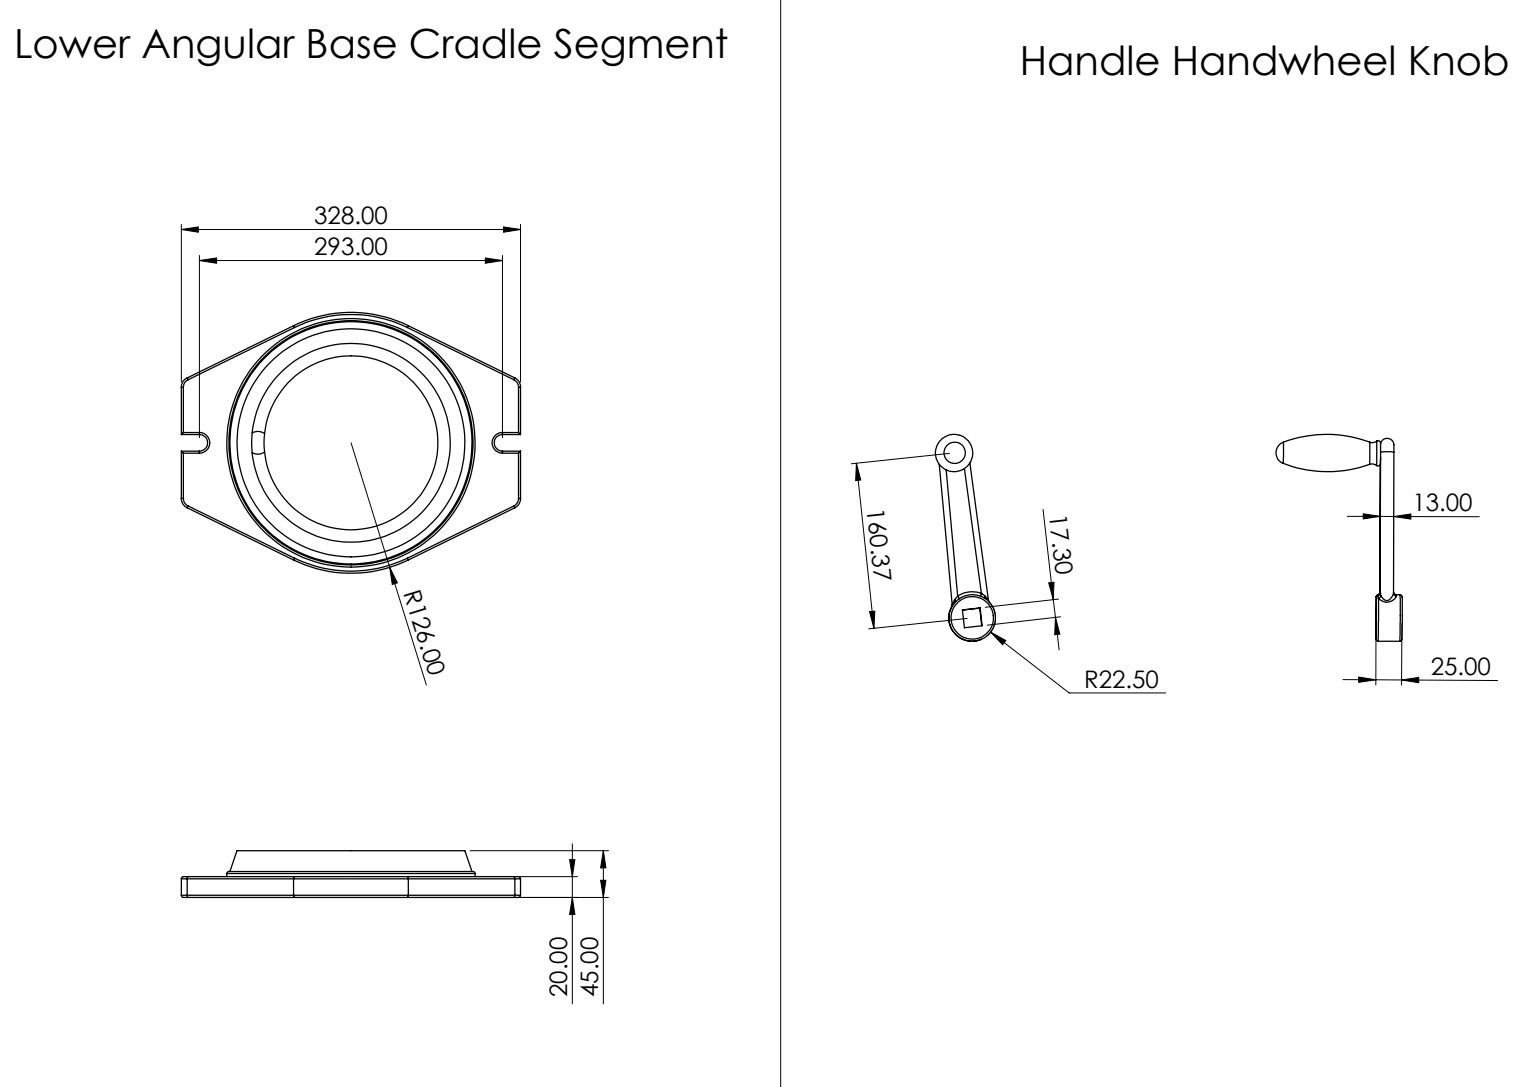
ISO-10303-21;
HEADER;
FILE_DESCRIPTION (('STEP AP214'),
    '1' );
FILE_NAME ('Lower Angular Base Cradle Segment.step',
    '2026-10-09T10:51:02',
    ( '' ),
    ( '' ),
    'SwSTEP 2.0',
    'SolidWorks 2026',
    '' );
FILE_SCHEMA (( 'AUTOMOTIVE_DESIGN' ));
ENDSEC;

DATA;
#11=AXIS2_PLACEMENT_3D ( 'NONE', #11203, #9587, #5900 ) ;
#14=ORIENTED_EDGE ( 'NONE', *, *, #14466, .T. ) ;
#36=VECTOR ( 'NONE', #11049, 1000.000000000000000 ) ;
#39=ORIENTED_EDGE ( 'NONE', *, *, #19350, .F. ) ;
#77=DIRECTION ( 'NONE',  ( 0.000000000000000000, 0.000000000000000000, -1.000000000000000000 ) ) ;
#83=DIRECTION ( 'NONE',  ( 0.000000000000000000, -1.000000000000000000, 0.000000000000000000 ) ) ;
#99=VERTEX_POINT ( 'NONE', #7105 ) ;
#118=EDGE_LOOP ( 'NONE', ( #17233, #4566 ) ) ;
#127=FACE_BOUND ( 'NONE', #21151, .T. ) ;
#139=ORIENTED_EDGE ( 'NONE', *, *, #21705, .T. ) ;
#155=EDGE_CURVE ( 'NONE', #11795, #1627, #509, .T. ) ;
#161=AXIS2_PLACEMENT_3D ( 'NONE', #9912, #15227, #6474 ) ;
#168=VERTEX_POINT ( 'NONE', #19161 ) ;
#170=EDGE_CURVE ( 'NONE', #168, #18579, #18934, .T. ) ;
#172=EDGE_CURVE ( 'NONE', #2811, #3408, #19534, .T. ) ;
#184=ORIENTED_EDGE ( 'NONE', *, *, #10599, .F. ) ;
#190=CIRCLE ( 'NONE', #9344, 2.000000000000000000 ) ;
#216=DIRECTION ( 'NONE',  ( 0.000000000000000000, 1.000000000000000000, -0.000000000000000000 ) ) ;
#237=DIRECTION ( 'NONE',  ( 0.000000000000000000, 0.000000000000000000, 1.000000000000000000 ) ) ;
#246=ORIENTED_EDGE ( 'NONE', *, *, #15979, .F. ) ;
#254=LINE ( 'NONE', #14055, #10043 ) ;
#259=DIRECTION ( 'NONE',  ( -0.000000000000000000, -1.000000000000000000, -0.000000000000000000 ) ) ;
#272=UNCERTAINTY_MEASURE_WITH_UNIT (LENGTH_MEASURE( 1.000000000000000082E-05 ), #22042, 'distance_accuracy_value', 'NONE');
#327=ORIENTED_EDGE ( 'NONE', *, *, #6954, .T. ) ;
#359=ORIENTED_EDGE ( 'NONE', *, *, #12423, .F. ) ;
#364=DIRECTION ( 'NONE',  ( -0.000000000000000000, -1.000000000000000000, 0.000000000000000000 ) ) ;
#443=VECTOR ( 'NONE', #5806, 1000.000000000000114 ) ;
#460=DIRECTION ( 'NONE',  ( 0.000000000000000000, 0.000000000000000000, 1.000000000000000000 ) ) ;
#465=AXIS2_PLACEMENT_3D ( 'NONE', #19858, #19338, #7694 ) ;
#466=AXIS2_PLACEMENT_3D ( 'NONE', #6505, #18462, #13187 ) ;
#468=DIRECTION ( 'NONE',  ( -0.000000000000000000, -1.000000000000000000, -0.000000000000000000 ) ) ;
#475=EDGE_CURVE ( 'NONE', #8008, #17969, #6839, .T. ) ;
#479=CIRCLE ( 'NONE', #8172, 10.00000000000001599 ) ;
#486=CARTESIAN_POINT ( 'NONE',  ( -164.0000000000000284, 19.17157287525381193, 8.000000000000019540 ) ) ;
#509=CIRCLE ( 'NONE', #21394, 8.000000000000003553 ) ;
#515=ORIENTED_EDGE ( 'NONE', *, *, #10366, .F. ) ;
#516=LINE ( 'NONE', #744, #20526 ) ;
#525=CARTESIAN_POINT ( 'NONE',  ( 163.9999999999992610, 1.999999999999998224, 53.76161406891480965 ) ) ;
#536=FACE_OUTER_BOUND ( 'NONE', #6630, .T. ) ;
#540=CARTESIAN_POINT ( 'NONE',  ( 161.9999999999998579, 0.000000000000000000, 10.00000000000220091 ) ) ;
#545=AXIS2_PLACEMENT_3D ( 'NONE', #10646, #3288, #5118 ) ;
#561=EDGE_CURVE ( 'NONE', #10233, #9740, #11615, .T. ) ;
#573=DIRECTION ( 'NONE',  ( 0.000000000000000000, -1.000000000000000000, 0.000000000000000000 ) ) ;
#576=CARTESIAN_POINT ( 'NONE',  ( -83.99999999999998579, 37.00000000000000711, 0.000000000000000000 ) ) ;
#585=EDGE_CURVE ( 'NONE', #7846, #1225, #20772, .T. ) ;
#605=DIRECTION ( 'NONE',  ( 0.000000000000000000, 0.000000000000000000, 1.000000000000000000 ) ) ;
#607=DIRECTION ( 'NONE',  ( -0.000000000000000000, -1.000000000000000000, 0.000000000000000000 ) ) ;
#614=ORIENTED_EDGE ( 'NONE', *, *, #21304, .F. ) ;
#619=ORIENTED_EDGE ( 'NONE', *, *, #6261, .F. ) ;
#620=ORIENTED_EDGE ( 'NONE', *, *, #15150, .T. ) ;
#632=EDGE_CURVE ( 'NONE', #17288, #1407, #18939, .T. ) ;
#636=EDGE_LOOP ( 'NONE', ( #1094, #22364, #825, #9647 ) ) ;
#643=CARTESIAN_POINT ( 'NONE',  ( -54.52327687265813694, 18.00000000000000355, 111.3697098814011781 ) ) ;
#654=DIRECTION ( 'NONE',  ( 0.000000000000000000, 0.000000000000000000, 1.000000000000000000 ) ) ;
#655=VECTOR ( 'NONE', #16102, 1000.000000000000000 ) ;
#660=CARTESIAN_POINT ( 'NONE',  ( 0.000000000000000000, 18.00000000000000355, 0.000000000000000000 ) ) ;
#669=EDGE_CURVE ( 'NONE', #4632, #17288, #3816, .T. ) ;
#671=ORIENTED_EDGE ( 'NONE', *, *, #11332, .T. ) ;
#673=AXIS2_PLACEMENT_3D ( 'NONE', #17290, #6819, #13736 ) ;
#688=CARTESIAN_POINT ( 'NONE',  ( 157.5176307659770885, 18.00000000000000355, -60.94675664190839370 ) ) ;
#695=CIRCLE ( 'NONE', #20840, 2.000000000000001332 ) ;
#706=ORIENTED_EDGE ( 'NONE', *, *, #11055, .F. ) ;
#724=VERTEX_POINT ( 'NONE', #1722 ) ;
#728=ORIENTED_EDGE ( 'NONE', *, *, #13180, .F. ) ;
#744=CARTESIAN_POINT ( 'NONE',  ( -146.5000000000000000, 20.00000000000000000, -7.999999999999981348 ) ) ;
#754=DIRECTION ( 'NONE',  ( -0.000000000000000000, -1.000000000000000000, -0.000000000000000000 ) ) ;
#756=DIRECTION ( 'NONE',  ( 0.8981428216242065554, 0.000000000000000000, 0.4397038457472354223 ) ) ;
#775=DIRECTION ( 'NONE',  ( 0.000000000000000000, 0.000000000000000000, -1.000000000000000000 ) ) ;
#777=DIRECTION ( 'NONE',  ( -1.000000000000000000, 0.000000000000000000, 0.000000000000000000 ) ) ;
#803=CARTESIAN_POINT ( 'NONE',  ( -164.0000000000000000, 18.00000000000000355, -53.76161406891256433 ) ) ;
#818=EDGE_CURVE ( 'NONE', #9599, #7572, #1748, .T. ) ;
#820=AXIS2_PLACEMENT_3D ( 'NONE', #8269, #17121, #15302 ) ;
#822=VERTEX_POINT ( 'NONE', #9641 ) ;
#825=ORIENTED_EDGE ( 'NONE', *, *, #1784, .F. ) ;
#827=AXIS2_PLACEMENT_3D ( 'NONE', #21475, #11159, #4013 ) ;
#867=DIRECTION ( 'NONE',  ( -0.8981428216242088869, 0.000000000000000000, 0.4397038457472309814 ) ) ;
#874=DIRECTION ( 'NONE',  ( 0.000000000000000000, 0.000000000000000000, -1.000000000000000000 ) ) ;
#893=DIRECTION ( 'NONE',  ( -0.000000000000000000, -1.000000000000000000, -0.000000000000000000 ) ) ;
#912=VECTOR ( 'NONE', #893, 1000.000000000000000 ) ;
#918=DIRECTION ( 'NONE',  ( 0.000000000000000000, -0.000000000000000000, 1.000000000000000000 ) ) ;
#924=LINE ( 'NONE', #16674, #12690 ) ;
#927=CARTESIAN_POINT ( 'NONE',  ( 1.236893267138826732E-14, 0.000000000000000000, 101.0000000000000000 ) ) ;
#955=DIRECTION ( 'NONE',  ( -0.000000000000000000, -1.000000000000000000, 0.000000000000000000 ) ) ;
#957=CARTESIAN_POINT ( 'NONE',  ( 162.0000000000000000, 1.999999999999998224, -2.262479907570350717E-12 ) ) ;
#966=CARTESIAN_POINT ( 'NONE',  ( -154.0000000000000000, 20.00000000000000000, -53.76161406891256433 ) ) ;
#972=CIRCLE ( 'NONE', #7187, 124.0000000000000000 ) ;
#977=DIRECTION ( 'NONE',  ( 0.4397038457472313144, 0.000000000000000000, -0.8981428216242086648 ) ) ;
#979=VERTEX_POINT ( 'NONE', #20950 ) ;
#982=ORIENTED_EDGE ( 'NONE', *, *, #22653, .T. ) ;
#1014=FACE_OUTER_BOUND ( 'NONE', #13248, .T. ) ;
#1018=VERTEX_POINT ( 'NONE', #4625 ) ;
#1025=DIRECTION ( 'NONE',  ( -1.000000000000000000, -0.000000000000000000, 9.912705577010318154E-17 ) ) ;
#1036=EDGE_LOOP ( 'NONE', ( #10873, #8707, #4402, #327 ) ) ;
#1044=DIRECTION ( 'NONE',  ( 0.000000000000000000, 1.000000000000000000, -0.000000000000000000 ) ) ;
#1047=DIRECTION ( 'NONE',  ( 0.000000000000000000, 0.000000000000000000, -1.000000000000000000 ) ) ;
#1050=DIRECTION ( 'NONE',  ( 0.8981428216242087759, -0.000000000000000000, -0.4397038457472309259 ) ) ;
#1052=DIRECTION ( 'NONE',  ( -0.000000000000000000, -1.000000000000000000, -0.000000000000000000 ) ) ;
#1055=DIRECTION ( 'NONE',  ( 1.458023040593674599E-16, 0.000000000000000000, 1.000000000000000000 ) ) ;
#1071=CYLINDRICAL_SURFACE ( 'NONE', #2276, 2.000000000000000000 ) ;
#1079=VECTOR ( 'NONE', #1276, 1000.000000000000000 ) ;
#1085=EDGE_CURVE ( 'NONE', #16346, #2665, #17059, .T. ) ;
#1090=CARTESIAN_POINT ( 'NONE',  ( 1.028703311283776507E-14, 45.00000000000000711, 83.99999999999998579 ) ) ;
#1094=ORIENTED_EDGE ( 'NONE', *, *, #6261, .T. ) ;
#1098=EDGE_CURVE ( 'NONE', #11124, #4632, #21172, .T. ) ;
#1102=ORIENTED_EDGE ( 'NONE', *, *, #1917, .T. ) ;
#1114=AXIS2_PLACEMENT_3D ( 'NONE', #8137, #15168, #22120 ) ;
#1154=CARTESIAN_POINT ( 'NONE',  ( -162.0000000000000000, 18.00000000000000355, -53.76161406891256433 ) ) ;
#1169=DIRECTION ( 'NONE',  ( -1.000000000000000000, 0.000000000000000000, 0.000000000000000000 ) ) ;
#1180=DIRECTION ( 'NONE',  ( -1.000000000000000000, 0.000000000000000000, 1.458023040593674599E-16 ) ) ;
#1181=CARTESIAN_POINT ( 'NONE',  ( 0.000000000000000000, 23.00000000000000000, 0.000000000000000000 ) ) ;
#1184=AXIS2_PLACEMENT_3D ( 'NONE', #9333, #5876, #12914 ) ;
#1185=DIRECTION ( 'NONE',  ( 0.000000000000000000, 0.000000000000000000, 1.000000000000000000 ) ) ;
#1192=CARTESIAN_POINT ( 'NONE',  ( 161.9999999999992610, 0.000000000000000000, 53.76161406891478123 ) ) ;
#1213=DIRECTION ( 'NONE',  ( -2.664535259100375697E-15, 0.000000000000000000, 1.000000000000000000 ) ) ;
#1214=CYLINDRICAL_SURFACE ( 'NONE', #18032, 2.000000000000001776 ) ;
#1225=VERTEX_POINT ( 'NONE', #3689 ) ;
#1241=EDGE_CURVE ( 'NONE', #1225, #14037, #18248, .T. ) ;
#1254=AXIS2_PLACEMENT_3D ( 'NONE', #3148, #17173, #10064 ) ;
#1269=DIRECTION ( 'NONE',  ( 2.449293598294706414E-16, 0.000000000000000000, 1.000000000000000000 ) ) ;
#1270=VECTOR ( 'NONE', #20131, 1000.000000000000000 ) ;
#1276=DIRECTION ( 'NONE',  ( -1.396592535537253658E-14, 0.000000000000000000, -1.000000000000000000 ) ) ;
#1282=ORIENTED_EDGE ( 'NONE', *, *, #11887, .F. ) ;
#1286=CARTESIAN_POINT ( 'NONE',  ( 54.52327687265659506, 20.00000000000000000, -111.3697098814019455 ) ) ;
#1288=VERTEX_POINT ( 'NONE', #2323 ) ;
#1296=CIRCLE ( 'NONE', #3486, 120.0000000000000000 ) ;
#1299=ADVANCED_FACE ( 'NONE', ( #19872 ), #18518, .F. ) ;
#1309=STYLED_ITEM ( 'NONE', ( #15085 ), #9845 ) ;
#1336=DIRECTION ( 'NONE',  ( 3.552713678800500929E-15, 0.000000000000000000, 1.000000000000000000 ) ) ;
#1339=DIRECTION ( 'NONE',  ( 1.000000000000000000, 0.000000000000000000, 1.372099599554301422E-14 ) ) ;
#1344=DIRECTION ( 'NONE',  ( -0.000000000000000000, -1.000000000000000000, -0.000000000000000000 ) ) ;
#1348=DIRECTION ( 'NONE',  ( 0.000000000000000000, 0.000000000000000000, -1.000000000000000000 ) ) ;
#1349=EDGE_CURVE ( 'NONE', #15641, #4119, #16444, .T. ) ;
#1350=ORIENTED_EDGE ( 'NONE', *, *, #13991, .F. ) ;
#1367=DIRECTION ( 'NONE',  ( 1.000000000000000000, -0.000000000000000000, -1.458023040593674599E-16 ) ) ;
#1375=DIRECTION ( 'NONE',  ( -0.000000000000000000, -1.000000000000000000, 0.000000000000000000 ) ) ;
#1380=CARTESIAN_POINT ( 'NONE',  ( 54.52327687265660927, 20.00000000000000000, 111.3697098814019029 ) ) ;
#1389=CARTESIAN_POINT ( 'NONE',  ( -164.0000000000000000, 18.00000000000000355, 0.000000000000000000 ) ) ;
#1392=ORIENTED_EDGE ( 'NONE', *, *, #10556, .F. ) ;
#1395=DIRECTION ( 'NONE',  ( 1.000000000000000000, 0.000000000000000000, 0.000000000000000000 ) ) ;
#1398=DIRECTION ( 'NONE',  ( 0.000000000000000000, 0.000000000000000000, -1.000000000000000000 ) ) ;
#1401=ORIENTED_EDGE ( 'NONE', *, *, #1478, .F. ) ;
#1407=VERTEX_POINT ( 'NONE', #22369 ) ;
#1431=EDGE_CURVE ( 'NONE', #1288, #17029, #10349, .T. ) ;
#1439=CIRCLE ( 'NONE', #6192, 78.99999999999998579 ) ;
#1440=ORIENTED_EDGE ( 'NONE', *, *, #17648, .T. ) ;
#1442=FACE_OUTER_BOUND ( 'NONE', #4234, .T. ) ;
#1443=DIRECTION ( 'NONE',  ( -0.000000000000000000, -1.000000000000000000, 0.000000000000000000 ) ) ;
#1478=EDGE_CURVE ( 'NONE', #9760, #979, #10929, .T. ) ;
#1501=EDGE_LOOP ( 'NONE', ( #17646, #17489, #7558, #20601, #8372, #14963, #15263, #20562, #9434, #13836, #9394, #3686, #8049, #16135, #18646, #21048, #4801, #16875, #2262, #19730, #15751 ) ) ;
#1519=AXIS2_PLACEMENT_3D ( 'NONE', #9593, #754, #11427 ) ;
#1522=EDGE_LOOP ( 'NONE', ( #6462, #16819, #9996, #12609 ) ) ;
#1523=EDGE_CURVE ( 'NONE', #9064, #5658, #4596, .T. ) ;
#1532=VERTEX_POINT ( 'NONE', #21232 ) ;
#1536=DIRECTION ( 'NONE',  ( 0.8981428216242028917, -0.000000000000000000, 0.4397038457472429718 ) ) ;
#1545=ORIENTED_EDGE ( 'NONE', *, *, #2061, .T. ) ;
#1550=VECTOR ( 'NONE', #4109, 1000.000000000000114 ) ;
#1551=EDGE_CURVE ( 'NONE', #9056, #6260, #1727, .T. ) ;
#1552=CARTESIAN_POINT ( 'NONE',  ( 0.000000000000000000, 25.00000000000000000, 0.000000000000000000 ) ) ;
#1554=PLANE ( 'NONE',  #3802 ) ;
#1558=CARTESIAN_POINT ( 'NONE',  ( 163.1715728752537018, 20.00000000000000355, -8.828427124748447596 ) ) ;
#1566=DIRECTION ( 'NONE',  ( 0.000000000000000000, 1.000000000000000000, 0.000000000000000000 ) ) ;
#1573=VECTOR ( 'NONE', #11501, 1000.000000000000000 ) ;
#1579=EDGE_LOOP ( 'NONE', ( #18293, #4104, #6095, #706 ) ) ;
#1580=CARTESIAN_POINT ( 'NONE',  ( 55.40268456415107323, 20.00000000000000000, -113.1659955246503557 ) ) ;
#1590=DIRECTION ( 'NONE',  ( 0.000000000000000000, 0.000000000000000000, 1.000000000000000000 ) ) ;
#1591=CARTESIAN_POINT ( 'NONE',  ( 157.5176307659770885, 20.00000000000000000, -60.94675664190840081 ) ) ;
#1604=ORIENTED_EDGE ( 'NONE', *, *, #10918, .T. ) ;
#1617=DIRECTION ( 'NONE',  ( 0.8981428216242088869, -0.000000000000000000, 0.4397038457472307593 ) ) ;
#1622=DIRECTION ( 'NONE',  ( 0.000000000000000000, -1.000000000000000000, 0.000000000000000000 ) ) ;
#1627=VERTEX_POINT ( 'NONE', #2968 ) ;
#1640=CARTESIAN_POINT ( 'NONE',  ( 0.000000000000000000, 45.00000000000000711, 0.000000000000000000 ) ) ;
#1660=CARTESIAN_POINT ( 'NONE',  ( -157.5176307659779411, 0.000000000000000000, 60.94675664190622655 ) ) ;
#1685=DIRECTION ( 'NONE',  ( -0.8981428216242028917, -0.000000000000000000, -0.4397038457472429718 ) ) ;
#1687=CARTESIAN_POINT ( 'NONE',  ( 0.000000000000000000, 20.00000000000000000, 0.000000000000000000 ) ) ;
#1693=CYLINDRICAL_SURFACE ( 'NONE', #7075, 8.000000000000003553 ) ;
#1714=DIRECTION ( 'NONE',  ( 0.000000000000000000, 0.000000000000000000, 1.000000000000000000 ) ) ;
#1721=DIRECTION ( 'NONE',  ( 0.000000000000000000, 0.000000000000000000, 1.000000000000000000 ) ) ;
#1722=CARTESIAN_POINT ( 'NONE',  ( 0.000000000000000000, 29.00000000000000711, -78.99999999999998579 ) ) ;
#1727=LINE ( 'NONE', #3893, #20440 ) ;
#1730=FACE_OUTER_BOUND ( 'NONE', #6402, .T. ) ;
#1742=EDGE_LOOP ( 'NONE', ( #11477, #2679, #19385, #12838 ) ) ;
#1748=CIRCLE ( 'NONE', #16801, 10.99999999999999289 ) ;
#1774=DIRECTION ( 'NONE',  ( -0.000000000000000000, -1.000000000000000000, -0.000000000000000000 ) ) ;
#1776=EDGE_CURVE ( 'NONE', #19048, #15773, #9846, .T. ) ;
#1782=AXIS2_PLACEMENT_3D ( 'NONE', #17932, #2168, #5721 ) ;
#1784=EDGE_CURVE ( 'NONE', #10110, #15773, #14258, .T. ) ;
#1786=DIRECTION ( 'NONE',  ( 1.000000000000000000, 0.000000000000000000, 0.000000000000000000 ) ) ;
#1794=ORIENTED_EDGE ( 'NONE', *, *, #18920, .F. ) ;
#1806=AXIS2_PLACEMENT_3D ( 'NONE', #5627, #7469, #5505 ) ;
#1808=DIRECTION ( 'NONE',  ( 0.000000000000000000, -1.000000000000000000, 0.000000000000000000 ) ) ;
#1809=DIRECTION ( 'NONE',  ( 0.000000000000000000, 0.000000000000000000, 1.000000000000000000 ) ) ;
#1829=EDGE_LOOP ( 'NONE', ( #4335, #17107, #8899, #14315, #21275, #17558, #10360, #7844, #3415, #6564 ) ) ;
#1831=ORIENTED_EDGE ( 'NONE', *, *, #20609, .T. ) ;
#1842=CIRCLE ( 'NONE', #13223, 101.0000000000000000 ) ;
#1852=CARTESIAN_POINT ( 'NONE',  ( 54.52327687265658085, 20.00000000000000000, -111.3697098814019171 ) ) ;
#1873=ORIENTED_EDGE ( 'NONE', *, *, #12470, .F. ) ;
#1879=VERTEX_POINT ( 'NONE', #21086 ) ;
#1909=AXIS2_PLACEMENT_3D ( 'NONE', #9756, #18257, #14830 ) ;
#1917=EDGE_CURVE ( 'NONE', #5531, #19256, #2593, .T. ) ;
#1926=CARTESIAN_POINT ( 'NONE',  ( -157.5176307659779127, 20.00000000000000000, 60.94675664190624786 ) ) ;
#1936=ADVANCED_FACE ( 'NONE', ( #536 ), #9602, .T. ) ;
#1971=CIRCLE ( 'NONE', #19570, 10.00000000000001599 ) ;
#1972=ORIENTED_EDGE ( 'NONE', *, *, #18630, .F. ) ;
#1975=FACE_OUTER_BOUND ( 'NONE', #9307, .T. ) ;
#1978=DIRECTION ( 'NONE',  ( -0.000000000000000000, -0.000000000000000000, 1.000000000000000000 ) ) ;
#1980=ADVANCED_FACE ( 'NONE', ( #20604 ), #15249, .T. ) ;
#1982=ORIENTED_EDGE ( 'NONE', *, *, #1431, .F. ) ;
#1991=VERTEX_POINT ( 'NONE', #18883 ) ;
#2000=EDGE_LOOP ( 'NONE', ( #18719, #17410, #7375, #11157 ) ) ;
#2003=AXIS2_PLACEMENT_3D ( 'NONE', #9292, #4227, #460 ) ;
#2011=ADVANCED_FACE ( 'NONE', ( #1442 ), #8422, .T. ) ;
#2028=DIRECTION ( 'NONE',  ( 0.000000000000000000, 0.000000000000000000, -1.000000000000000000 ) ) ;
#2030=ORIENTED_EDGE ( 'NONE', *, *, #6944, .T. ) ;
#2034=ADVANCED_FACE ( 'NONE', ( #4971 ), #12001, .T. ) ;
#2061=EDGE_CURVE ( 'NONE', #10705, #9211, #22294, .T. ) ;
#2069=EDGE_CURVE ( 'NONE', #21740, #9403, #15804, .T. ) ;
#2089=ADVANCED_FACE ( 'NONE', ( #12577 ), #8646, .F. ) ;
#2096=DIRECTION ( 'NONE',  ( 0.000000000000000000, 0.000000000000000000, 1.000000000000000000 ) ) ;
#2101=LINE ( 'NONE', #1660, #12535 ) ;
#2103=ORIENTED_EDGE ( 'NONE', *, *, #18624, .T. ) ;
#2106=ORIENTED_EDGE ( 'NONE', *, *, #19715, .T. ) ;
#2130=CARTESIAN_POINT ( 'NONE',  ( 146.5000000000000000, 20.00000000000000000, -2.025191382850354537E-12 ) ) ;
#2134=VERTEX_POINT ( 'NONE', #8879 ) ;
#2137=PRODUCT_DEFINITION ( 'UNKNOWN', '', #8434, #18911 ) ;
#2153=ORIENTED_EDGE ( 'NONE', *, *, #21573, .T. ) ;
#2156=AXIS2_PLACEMENT_3D ( 'NONE', #8737, #13938, #14184 ) ;
#2168=DIRECTION ( 'NONE',  ( 0.000000000000000000, 1.000000000000000000, -0.000000000000000000 ) ) ;
#2184=LINE ( 'NONE', #21035, #3366 ) ;
#2207=AXIS2_PLACEMENT_3D ( 'NONE', #18108, #11544, #7746 ) ;
#2218=AXIS2_PLACEMENT_3D ( 'NONE', #6057, #13192, #15152 ) ;
#2223=DIRECTION ( 'NONE',  ( 0.000000000000000000, 0.000000000000000000, 1.000000000000000000 ) ) ;
#2224=CYLINDRICAL_SURFACE ( 'NONE', #10412, 2.000000000000004441 ) ;
#2239=EDGE_CURVE ( 'NONE', #3243, #7424, #19014, .T. ) ;
#2247=CIRCLE ( 'NONE', #11065, 2.000000000000000000 ) ;
#2261=DIRECTION ( 'NONE',  ( 0.000000000000000000, 1.000000000000000000, -0.000000000000000000 ) ) ;
#2262=ORIENTED_EDGE ( 'NONE', *, *, #10736, .T. ) ;
#2272=ORIENTED_EDGE ( 'NONE', *, *, #5577, .T. ) ;
#2276=AXIS2_PLACEMENT_3D ( 'NONE', #15101, #6359, #20355 ) ;
#2282=CARTESIAN_POINT ( 'NONE',  ( -158.3970384574724051, 18.00000000000000355, 62.74304228515463677 ) ) ;
#2293=DIRECTION ( 'NONE',  ( 0.4397038457472340900, 0.000000000000000000, -0.8981428216242072216 ) ) ;
#2297=CARTESIAN_POINT ( 'NONE',  ( -101.0000000000000000, 29.00000000000000355, 9.420035382405126825E-16 ) ) ;
#2307=CARTESIAN_POINT ( 'NONE',  ( -162.0000000000000000, 18.00000000000000355, 3.967855629237424480E-14 ) ) ;
#2316=AXIS2_PLACEMENT_3D ( 'NONE', #8607, #13906, #237 ) ;
#2323=CARTESIAN_POINT ( 'NONE',  ( 157.5176307659771169, 0.000000000000000000, 60.94675664190834397 ) ) ;
#2327=DIRECTION ( 'NONE',  ( 0.000000000000000000, 0.000000000000000000, -1.000000000000000000 ) ) ;
#2334=ORIENTED_EDGE ( 'NONE', *, *, #172, .F. ) ;
#2360=ORIENTED_EDGE ( 'NONE', *, *, #21029, .F. ) ;
#2382=AXIS2_PLACEMENT_3D ( 'NONE', #19722, #16437, #3785 ) ;
#2389=ORIENTED_EDGE ( 'NONE', *, *, #15150, .F. ) ;
#2412=VECTOR ( 'NONE', #10464, 1000.000000000000000 ) ;
#2426=ORIENTED_EDGE ( 'NONE', *, *, #4092, .T. ) ;
#2428=ORIENTED_EDGE ( 'NONE', *, *, #22655, .T. ) ;
#2456=DIRECTION ( 'NONE',  ( 0.000000000000000000, 0.000000000000000000, 1.000000000000000000 ) ) ;
#2461=CARTESIAN_POINT ( 'NONE',  ( 55.40268456415105902, 1.999999999999998224, -113.1659955246503699 ) ) ;
#2469=VERTEX_POINT ( 'NONE', #15654 ) ;
#2506=DIRECTION ( 'NONE',  ( -0.000000000000000000, -1.000000000000000000, 0.000000000000000000 ) ) ;
#2508=CIRCLE ( 'NONE', #7273, 83.99999999999998579 ) ;
#2514=DIRECTION ( 'NONE',  ( 0.000000000000000000, 1.000000000000000000, 0.000000000000000000 ) ) ;
#2528=ADVANCED_FACE ( 'NONE', ( #5844 ), #5968, .T. ) ;
#2532=ORIENTED_EDGE ( 'NONE', *, *, #12333, .F. ) ;
#2537=( BOUNDED_CURVE ( )  B_SPLINE_CURVE ( 3, ( #10708, #5746, #486, #3914 ),
 .UNSPECIFIED., .F., .T. ) 
 B_SPLINE_CURVE_WITH_KNOTS ( ( 4, 4 ),
 ( 1.570796326794896558, 3.141592653589793116 ),
 .UNSPECIFIED. ) 
 CURVE ( )  GEOMETRIC_REPRESENTATION_ITEM ( )  RATIONAL_B_SPLINE_CURVE ( ( 1.000000000000000000, 0.8047378541243649375, 0.8047378541243649375, 1.000000000000000000 ) ) 
 REPRESENTATION_ITEM ( '' )  );
#2544=ORIENTED_EDGE ( 'NONE', *, *, #19748, .T. ) ;
#2552=LINE ( 'NONE', #18082, #11928 ) ;
#2566=CIRCLE ( 'NONE', #4001, 96.00000000000000000 ) ;
#2573=FACE_OUTER_BOUND ( 'NONE', #1501, .T. ) ;
#2574=CARTESIAN_POINT ( 'NONE',  ( 146.4999999999998579, 0.000000000000000000, 10.00000000000199130 ) ) ;
#2581=AXIS2_PLACEMENT_3D ( 'NONE', #12804, #21729, #14437 ) ;
#2586=CARTESIAN_POINT ( 'NONE',  ( -55.40268456415264353, 1.999999999999998224, -113.1659955246495883 ) ) ;
#2593=LINE ( 'NONE', #7536, #20472 ) ;
#2595=VECTOR ( 'NONE', #19673, 1000.000000000000000 ) ;
#2616=CIRCLE ( 'NONE', #9940, 2.000000000000001776 ) ;
#2618=AXIS2_PLACEMENT_3D ( 'NONE', #22365, #10006, #4809 ) ;
#2620=CARTESIAN_POINT ( 'NONE',  ( 0.000000000000000000, 0.000000000000000000, 0.000000000000000000 ) ) ;
#2621=ADVANCED_FACE ( 'NONE', ( #4120 ), #3899, .T. ) ;
#2624=CARTESIAN_POINT ( 'NONE',  ( 146.4999999999998579, 0.000000000000000000, -10.00000000000202860 ) ) ;
#2633=DIRECTION ( 'NONE',  ( 0.000000000000000000, 1.000000000000000000, -0.000000000000000000 ) ) ;
#2645=DIRECTION ( 'NONE',  ( -1.000000000000000000, 0.000000000000000000, 0.000000000000000000 ) ) ;
#2650=EDGE_CURVE ( 'NONE', #9740, #19048, #18597, .T. ) ;
#2652=CARTESIAN_POINT ( 'NONE',  ( 0.000000000000000000, 18.00000000000000355, 0.000000000000000000 ) ) ;
#2658=FACE_OUTER_BOUND ( 'NONE', #17459, .T. ) ;
#2665=VERTEX_POINT ( 'NONE', #7812 ) ;
#2670=AXIS2_PLACEMENT_3D ( 'NONE', #6925, #14618, #7050 ) ;
#2674=DIRECTION ( 'NONE',  ( -0.000000000000000000, -1.000000000000000000, -0.000000000000000000 ) ) ;
#2679=ORIENTED_EDGE ( 'NONE', *, *, #19298, .F. ) ;
#2683=( BOUNDED_CURVE ( )  B_SPLINE_CURVE ( 3, ( #12861, #7800, #5720, #16550 ),
 .UNSPECIFIED., .F., .T. ) 
 B_SPLINE_CURVE_WITH_KNOTS ( ( 4, 4 ),
 ( 4.712388980384689674, 6.283185307179586232 ),
 .UNSPECIFIED. ) 
 CURVE ( )  GEOMETRIC_REPRESENTATION_ITEM ( )  RATIONAL_B_SPLINE_CURVE ( ( 1.000000000000000000, 0.8047378541243649375, 0.8047378541243649375, 1.000000000000000000 ) ) 
 REPRESENTATION_ITEM ( '' )  );
#2689=EDGE_CURVE ( 'NONE', #8292, #21383, #21901, .T. ) ;
#2690=FACE_OUTER_BOUND ( 'NONE', #20598, .T. ) ;
#2694=ORIENTED_EDGE ( 'NONE', *, *, #11745, .F. ) ;
#2696=FACE_OUTER_BOUND ( 'NONE', #21989, .T. ) ;
#2699=CARTESIAN_POINT ( 'NONE',  ( 54.52327687265658085, 18.00000000000000355, -111.3697098814019171 ) ) ;
#2707=LINE ( 'NONE', #6142, #1270 ) ;
#2711=ORIENTED_EDGE ( 'NONE', *, *, #16561, .F. ) ;
#2726=VECTOR ( 'NONE', #1050, 1000.000000000000114 ) ;
#2736=CARTESIAN_POINT ( 'NONE',  ( -164.0000000000000000, 20.00000000000000000, 0.000000000000000000 ) ) ;
#2739=FACE_OUTER_BOUND ( 'NONE', #22266, .T. ) ;
#2751=EDGE_CURVE ( 'NONE', #11917, #7779, #4721, .T. ) ;
#2767=CARTESIAN_POINT ( 'NONE',  ( 146.4999999999998863, 20.00000000000000000, 8.000000000001989520 ) ) ;
#2781=ORIENTED_EDGE ( 'NONE', *, *, #2751, .F. ) ;
#2794=EDGE_CURVE ( 'NONE', #22165, #19122, #2972, .T. ) ;
#2798=FACE_OUTER_BOUND ( 'NONE', #20156, .T. ) ;
#2811=VERTEX_POINT ( 'NONE', #1380 ) ;
#2812=DIRECTION ( 'NONE',  ( 0.000000000000000000, 0.000000000000000000, -1.000000000000000000 ) ) ;
#2832=EDGE_CURVE ( 'NONE', #5236, #822, #17460, .T. ) ;
#2837=VERTEX_POINT ( 'NONE', #14005 ) ;
#2846=FACE_OUTER_BOUND ( 'NONE', #10676, .T. ) ;
#2856=CARTESIAN_POINT ( 'NONE',  ( 0.000000000000000000, 37.00000000000000711, 0.000000000000000000 ) ) ;
#2859=DIRECTION ( 'NONE',  ( -1.000000000000000000, -0.000000000000000000, -0.000000000000000000 ) ) ;
#2865=ORIENTED_EDGE ( 'NONE', *, *, #17744, .F. ) ;
#2873=LINE ( 'NONE', #11721, #21268 ) ;
#2874=ORIENTED_EDGE ( 'NONE', *, *, #6944, .F. ) ;
#2892=EDGE_CURVE ( 'NONE', #12157, #8554, #13779, .T. ) ;
#2916=VERTEX_POINT ( 'NONE', #10442 ) ;
#2917=AXIS2_PLACEMENT_3D ( 'NONE', #1580, #20400, #13867 ) ;
#2919=CARTESIAN_POINT ( 'NONE',  ( -55.40268456415262932, 20.00000000000000000, 113.1659955246495883 ) ) ;
#2925=CARTESIAN_POINT ( 'NONE',  ( 0.000000000000000000, 0.000000000000000000, -78.99999999999998579 ) ) ;
#2928=FACE_OUTER_BOUND ( 'NONE', #1579, .T. ) ;
#2933=DIRECTION ( 'NONE',  ( -0.000000000000000000, -1.000000000000000000, -0.000000000000000000 ) ) ;
#2951=EDGE_CURVE ( 'NONE', #12157, #19445, #4786, .T. ) ;
#2955=VERTEX_POINT ( 'NONE', #5013 ) ;
#2961=CARTESIAN_POINT ( 'NONE',  ( 163.9999999999998863, 18.00000000000000355, 8.000000000002229328 ) ) ;
#2965=CARTESIAN_POINT ( 'NONE',  ( -164.0000000000000000, 20.00000000000000000, 53.76161406891260697 ) ) ;
#2968=CARTESIAN_POINT ( 'NONE',  ( -146.5000000000000000, 1.999999999999998224, 8.000000000000017764 ) ) ;
#2972=LINE ( 'NONE', #9987, #6926 ) ;
#2992=SURFACE_STYLE_USAGE ( .BOTH. , #9679 ) ;
#2995=AXIS2_PLACEMENT_3D ( 'NONE', #14715, #2633, #12992 ) ;
#3011=EDGE_CURVE ( 'NONE', #14045, #1288, #12477, .T. ) ;
#3013=AXIS2_PLACEMENT_3D ( 'NONE', #8562, #5101, #10300 ) ;
#3023=ORIENTED_EDGE ( 'NONE', *, *, #19180, .F. ) ;
#3030=VECTOR ( 'NONE', #19503, 1000.000000000000000 ) ;
#3032=ORIENTED_EDGE ( 'NONE', *, *, #13991, .T. ) ;
#3042=FACE_OUTER_BOUND ( 'NONE', #12897, .T. ) ;
#3048=AXIS2_PLACEMENT_3D ( 'NONE', #15582, #22532, #4864 ) ;
#3075=FACE_OUTER_BOUND ( 'NONE', #4265, .T. ) ;
#3085=CARTESIAN_POINT ( 'NONE',  ( 0.000000000000000000, 45.00000000000000711, -83.99999999999998579 ) ) ;
#3102=CARTESIAN_POINT ( 'NONE',  ( 0.000000000000000000, 0.000000000000000000, 0.000000000000000000 ) ) ;
#3128=ORIENTED_EDGE ( 'NONE', *, *, #1349, .F. ) ;
#3129=ORIENTED_EDGE ( 'NONE', *, *, #22301, .F. ) ;
#3135=( NAMED_UNIT ( * ) SI_UNIT ( $, .STERADIAN. ) SOLID_ANGLE_UNIT ( ) );
#3141=EDGE_CURVE ( 'NONE', #18838, #9416, #12211, .T. ) ;
#3148=CARTESIAN_POINT ( 'NONE',  ( -146.5000000000000000, 18.00000000000000355, 2.081668171172168513E-14 ) ) ;
#3149=EDGE_CURVE ( 'NONE', #10602, #22152, #21465, .T. ) ;
#3152=CARTESIAN_POINT ( 'NONE',  ( 1.445083222993876641E-14, 23.00000000000000000, -118.0000000000000000 ) ) ;
#3153=CARTESIAN_POINT ( 'NONE',  ( -90.00000000000000000, 45.00100000000000477, 10.99999999999999289 ) ) ;
#3178=DIRECTION ( 'NONE',  ( 0.000000000000000000, 0.000000000000000000, -1.000000000000000000 ) ) ;
#3180=DIRECTION ( 'NONE',  ( -1.000000000000000000, 0.000000000000000000, -1.362186893977296347E-14 ) ) ;
#3181=ADVANCED_FACE ( 'NONE', ( #19629 ), #11024, .T. ) ;
#3191=CARTESIAN_POINT ( 'NONE',  ( -55.40268456415265774, 18.00000000000000355, -113.1659955246495741 ) ) ;
#3196=CARTESIAN_POINT ( 'NONE',  ( -1.386679829960242619E-13, 20.00000000000000000, -9.999999999999994671 ) ) ;
#3217=ORIENTED_EDGE ( 'NONE', *, *, #1523, .F. ) ;
#3224=CARTESIAN_POINT ( 'NONE',  ( 146.4999999999998579, 20.00000000000000000, -10.00000000000202682 ) ) ;
#3243=VERTEX_POINT ( 'NONE', #18490 ) ;
#3246=ORIENTED_EDGE ( 'NONE', *, *, #6278, .F. ) ;
#3252=EDGE_CURVE ( 'NONE', #15219, #6364, #20313, .T. ) ;
#3254=VERTEX_POINT ( 'NONE', #11599 ) ;
#3267=ORIENTED_EDGE ( 'NONE', *, *, #818, .T. ) ;
#3276=CARTESIAN_POINT ( 'NONE',  ( 0.000000000000000000, 25.00000000000000000, -120.0000000000000000 ) ) ;
#3283=EDGE_CURVE ( 'NONE', #1879, #2134, #2566, .T. ) ;
#3288=DIRECTION ( 'NONE',  ( 0.000000000000000000, 1.000000000000000000, -0.000000000000000000 ) ) ;
#3298=DIRECTION ( 'NONE',  ( 0.4397038457472313144, 0.000000000000000000, -0.8981428216242086648 ) ) ;
#3310=CARTESIAN_POINT ( 'NONE',  ( 54.52327687265660927, 18.00000000000000355, 111.3697098814019029 ) ) ;
#3312=DIRECTION ( 'NONE',  ( 0.000000000000000000, 0.000000000000000000, -1.000000000000000000 ) ) ;
#3320=EDGE_LOOP ( 'NONE', ( #19313, #16483, #19262, #6872 ) ) ;
#3325=AXIS2_PLACEMENT_3D ( 'NONE', #11563, #18784, #12008 ) ;
#3348=VERTEX_POINT ( 'NONE', #3085 ) ;
#3349=DIRECTION ( 'NONE',  ( -0.000000000000000000, -1.000000000000000000, -0.000000000000000000 ) ) ;
#3350=AXIS2_PLACEMENT_3D ( 'NONE', #10883, #17909, #7433 ) ;
#3361=DIRECTION ( 'NONE',  ( 1.000000000000000000, 0.000000000000000000, 1.387778780781445676E-14 ) ) ;
#3363=DIRECTION ( 'NONE',  ( 0.000000000000000000, 1.000000000000000000, -0.000000000000000000 ) ) ;
#3366=VECTOR ( 'NONE', #5287, 1000.000000000000000 ) ;
#3368=AXIS2_PLACEMENT_3D ( 'NONE', #5009, #8347, #22339 ) ;
#3378=VECTOR ( 'NONE', #6174, 1000.000000000000000 ) ;
#3408=VERTEX_POINT ( 'NONE', #13883 ) ;
#3411=ORIENTED_EDGE ( 'NONE', *, *, #13888, .T. ) ;
#3415=ORIENTED_EDGE ( 'NONE', *, *, #12655, .F. ) ;
#3423=AXIS2_PLACEMENT_3D ( 'NONE', #20142, #7977, #4414 ) ;
#3432=DIRECTION ( 'NONE',  ( 1.000000000000000000, 0.000000000000000000, -9.912705577010318154E-17 ) ) ;
#3439=DIRECTION ( 'NONE',  ( -3.987059982602682030E-17, -0.9455185755993167351, -0.3255681544571568109 ) ) ;
#3450=PLANE ( 'NONE',  #2316 ) ;
#3451=DIRECTION ( 'NONE',  ( -0.4397038457472424167, 0.000000000000000000, -0.8981428216242032248 ) ) ;
#3485=EDGE_LOOP ( 'NONE', ( #7503, #21513, #17440, #14077 ) ) ;
#3486=AXIS2_PLACEMENT_3D ( 'NONE', #1181, #16592, #20220 ) ;
#3492=ORIENTED_EDGE ( 'NONE', *, *, #10051, .F. ) ;
#3495=CARTESIAN_POINT ( 'NONE',  ( -154.0000000000000000, 0.000000000000000000, 53.76161406891259986 ) ) ;
#3496=CARTESIAN_POINT ( 'NONE',  ( 1.469576158976823671E-14, 23.00000000000000000, 120.0000000000000000 ) ) ;
#3529=VERTEX_POINT ( 'NONE', #21652 ) ;
#3546=CARTESIAN_POINT ( 'NONE',  ( 157.5176307659771169, 20.00000000000000000, 60.94675664190834397 ) ) ;
#3547=DIRECTION ( 'NONE',  ( 0.000000000000000000, 1.000000000000000000, -0.000000000000000000 ) ) ;
#3569=CARTESIAN_POINT ( 'NONE',  ( 161.9999999999998579, 0.000000000000000000, 10.00000000000220091 ) ) ;
#3596=EDGE_CURVE ( 'NONE', #7779, #21740, #21595, .T. ) ;
#3607=VECTOR ( 'NONE', #16039, 1000.000000000000000 ) ;
#3632=VECTOR ( 'NONE', #20078, 1000.000000000000000 ) ;
#3634=LINE ( 'NONE', #10647, #14284 ) ;
#3652=DIRECTION ( 'NONE',  ( 0.000000000000000000, 0.000000000000000000, 1.000000000000000000 ) ) ;
#3653=DIRECTION ( 'NONE',  ( 0.8981428216242027807, 0.000000000000000000, -0.4397038457472431938 ) ) ;
#3659=VERTEX_POINT ( 'NONE', #5756 ) ;
#3666=DIRECTION ( 'NONE',  ( 0.000000000000000000, 0.000000000000000000, 1.000000000000000000 ) ) ;
#3682=CARTESIAN_POINT ( 'NONE',  ( -1.386679829960242619E-13, 2.000000000000000000, -9.999999999999994671 ) ) ;
#3686=ORIENTED_EDGE ( 'NONE', *, *, #2069, .T. ) ;
#3689=CARTESIAN_POINT ( 'NONE',  ( 3.086109933851330151E-14, 1.999999999999998224, 126.0000000000000000 ) ) ;
#3734=EDGE_LOOP ( 'NONE', ( #9958, #4107 ) ) ;
#3738=ADVANCED_FACE ( 'NONE', ( #14876 ), #21817, .T. ) ;
#3743=EDGE_CURVE ( 'NONE', #11172, #2955, #20824, .T. ) ;
#3768=VECTOR ( 'NONE', #14937, 1000.000000000000114 ) ;
#3772=EDGE_LOOP ( 'NONE', ( #2103, #9863, #21778, #6767 ) ) ;
#3783=DIRECTION ( 'NONE',  ( 0.000000000000000000, 0.000000000000000000, -1.000000000000000000 ) ) ;
#3785=DIRECTION ( 'NONE',  ( 0.000000000000000000, 0.000000000000000000, 1.000000000000000000 ) ) ;
#3788=VECTOR ( 'NONE', #18661, 1000.000000000000000 ) ;
#3789=AXIS2_PLACEMENT_3D ( 'NONE', #15759, #10684, #5378 ) ;
#3798=ADVANCED_FACE ( 'NONE', ( #6671 ), #14248, .T. ) ;
#3802=AXIS2_PLACEMENT_3D ( 'NONE', #10510, #7274, #7170 ) ;
#3809=ORIENTED_EDGE ( 'NONE', *, *, #2794, .F. ) ;
#3816=CIRCLE ( 'NONE', #16679, 8.000000000000003553 ) ;
#3832=DIRECTION ( 'NONE',  ( 1.000000000000000000, 0.000000000000000000, -1.387778780781445833E-14 ) ) ;
#3835=ORIENTED_EDGE ( 'NONE', *, *, #3149, .T. ) ;
#3862=ORIENTED_EDGE ( 'NONE', *, *, #3596, .F. ) ;
#3880=ADVANCED_FACE ( 'NONE', ( #13526 ), #20839, .T. ) ;
#3893=CARTESIAN_POINT ( 'NONE',  ( 55.40268456415105902, 20.00000000000000000, -113.1659955246503699 ) ) ;
#3899=CYLINDRICAL_SURFACE ( 'NONE', #3982, 2.000000000000001332 ) ;
#3903=ORIENTED_EDGE ( 'NONE', *, *, #3283, .F. ) ;
#3906=LINE ( 'NONE', #14270, #21683 ) ;
#3908=CARTESIAN_POINT ( 'NONE',  ( 153.9999999999992610, 18.00000000000000355, -53.76161406891471017 ) ) ;
#3911=ORIENTED_EDGE ( 'NONE', *, *, #6131, .F. ) ;
#3914=CARTESIAN_POINT ( 'NONE',  ( -164.0000000000000000, 18.00000000000000355, 8.000000000000019540 ) ) ;
#3937=VERTEX_POINT ( 'NONE', #13857 ) ;
#3967=DIRECTION ( 'NONE',  ( 0.4397038457472424167, 0.000000000000000000, -0.8981428216242032248 ) ) ;
#3982=AXIS2_PLACEMENT_3D ( 'NONE', #9058, #11260, #18269 ) ;
#3989=FACE_OUTER_BOUND ( 'NONE', #10763, .T. ) ;
#3994=ORIENTED_EDGE ( 'NONE', *, *, #17938, .T. ) ;
#4001=AXIS2_PLACEMENT_3D ( 'NONE', #2856, #15179, #18821 ) ;
#4002=ORIENTED_EDGE ( 'NONE', *, *, #21675, .T. ) ;
#4010=EDGE_LOOP ( 'NONE', ( #2428, #19590, #9387, #16670 ) ) ;
#4013=DIRECTION ( 'NONE',  ( 0.000000000000000000, 0.000000000000000000, 1.000000000000000000 ) ) ;
#4024=DIRECTION ( 'NONE',  ( 0.000000000000000000, 1.000000000000000000, -0.000000000000000000 ) ) ;
#4042=CARTESIAN_POINT ( 'NONE',  ( -146.5000000000000000, 1.999999999999998224, -7.999999999999981348 ) ) ;
#4045=ADVANCED_FACE ( 'NONE', ( #6254 ), #17189, .T. ) ;
#4052=CARTESIAN_POINT ( 'NONE',  ( -162.0000000000000000, 0.000000000000000000, -53.76161406891256433 ) ) ;
#4064=ORIENTED_EDGE ( 'NONE', *, *, #13445, .F. ) ;
#4075=CARTESIAN_POINT ( 'NONE',  ( 163.9999999999998295, 0.8284271247461892917, -8.000000000002268408 ) ) ;
#4088=ORIENTED_EDGE ( 'NONE', *, *, #17676, .F. ) ;
#4092=EDGE_CURVE ( 'NONE', #822, #10707, #695, .T. ) ;
#4102=LINE ( 'NONE', #5479, #3030 ) ;
#4104=ORIENTED_EDGE ( 'NONE', *, *, #9891, .F. ) ;
#4107=ORIENTED_EDGE ( 'NONE', *, *, #4169, .F. ) ;
#4109=DIRECTION ( 'NONE',  ( 0.8981428216242087759, -0.000000000000000000, -0.4397038457472309259 ) ) ;
#4115=DIRECTION ( 'NONE',  ( 0.000000000000000000, 1.000000000000000000, -0.000000000000000000 ) ) ;
#4116=CIRCLE ( 'NONE', #8892, 2.000000000000001776 ) ;
#4119=VERTEX_POINT ( 'NONE', #2586 ) ;
#4120=FACE_OUTER_BOUND ( 'NONE', #13840, .T. ) ;
#4141=DIRECTION ( 'NONE',  ( 0.000000000000000000, 0.000000000000000000, -1.000000000000000000 ) ) ;
#4155=AXIS2_PLACEMENT_3D ( 'NONE', #3682, #15780, #14403 ) ;
#4158=AXIS2_PLACEMENT_3D ( 'NONE', #12119, #12464, #8882 ) ;
#4168=CARTESIAN_POINT ( 'NONE',  ( 0.000000000000000000, 29.00000000000000355, -101.0000000000000000 ) ) ;
#4169=EDGE_CURVE ( 'NONE', #9064, #3348, #2508, .T. ) ;
#4175=AXIS2_PLACEMENT_3D ( 'NONE', #10513, #3547, #10673 ) ;
#4198=CARTESIAN_POINT ( 'NONE',  ( 163.9999999999992610, 18.00000000000000355, 53.76161406891480965 ) ) ;
#4205=AXIS2_PLACEMENT_3D ( 'NONE', #14508, #5729, #11029 ) ;
#4227=DIRECTION ( 'NONE',  ( 0.000000000000000000, 1.000000000000000000, -0.000000000000000000 ) ) ;
#4231=ORIENTED_EDGE ( 'NONE', *, *, #13180, .T. ) ;
#4233=DIRECTION ( 'NONE',  ( 0.4397038457472424167, 0.000000000000000000, 0.8981428216242032248 ) ) ;
#4234=EDGE_LOOP ( 'NONE', ( #5445, #11256, #17197, #20029 ) ) ;
#4239=CIRCLE ( 'NONE', #21836, 10.99999999999999289 ) ;
#4242=EDGE_CURVE ( 'NONE', #14514, #9599, #6234, .T. ) ;
#4247=DIRECTION ( 'NONE',  ( 0.000000000000000000, 0.000000000000000000, 1.000000000000000000 ) ) ;
#4252=FACE_OUTER_BOUND ( 'NONE', #5112, .T. ) ;
#4257=DIRECTION ( 'NONE',  ( -1.000000000000000000, 0.000000000000000000, 2.449293598294706414E-16 ) ) ;
#4258=FACE_OUTER_BOUND ( 'NONE', #14598, .T. ) ;
#4265=EDGE_LOOP ( 'NONE', ( #6241, #9467, #18304, #5417 ) ) ;
#4268=( BOUNDED_CURVE ( )  B_SPLINE_CURVE ( 3, ( #21207, #9263, #9024, #14578 ),
 .UNSPECIFIED., .F., .T. ) 
 B_SPLINE_CURVE_WITH_KNOTS ( ( 4, 4 ),
 ( 3.141592653589793116, 4.712388980384689674 ),
 .UNSPECIFIED. ) 
 CURVE ( )  GEOMETRIC_REPRESENTATION_ITEM ( )  RATIONAL_B_SPLINE_CURVE ( ( 1.000000000000000000, 0.8047378541243649375, 0.8047378541243649375, 1.000000000000000000 ) ) 
 REPRESENTATION_ITEM ( '' )  );
#4290=AXIS2_PLACEMENT_3D ( 'NONE', #13494, #3361, #6802 ) ;
#4315=AXIS2_PLACEMENT_3D ( 'NONE', #10236, #22267, #1185 ) ;
#4327=ORIENTED_EDGE ( 'NONE', *, *, #17265, .F. ) ;
#4329=ORIENTED_EDGE ( 'NONE', *, *, #16427, .F. ) ;
#4335=ORIENTED_EDGE ( 'NONE', *, *, #9920, .F. ) ;
#4338=EDGE_CURVE ( 'NONE', #7424, #7803, #15375, .T. ) ;
#4342=DIRECTION ( 'NONE',  ( 0.000000000000000000, 0.000000000000000000, -1.000000000000000000 ) ) ;
#4351=FACE_OUTER_BOUND ( 'NONE', #6537, .T. ) ;
#4354=CARTESIAN_POINT ( 'NONE',  ( 0.000000000000000000, 29.00000000000000711, 0.000000000000000000 ) ) ;
#4356=ORIENTED_EDGE ( 'NONE', *, *, #18920, .T. ) ;
#4366=DIRECTION ( 'NONE',  ( 8.881784197001252323E-16, 0.000000000000000000, 1.000000000000000000 ) ) ;
#4370=DIRECTION ( 'NONE',  ( -0.000000000000000000, 0.000000000000000000, 1.000000000000000000 ) ) ;
#4371=ADVANCED_FACE ( 'NONE', ( #19985 ), #11274, .F. ) ;
#4378=ORIENTED_EDGE ( 'NONE', *, *, #6433, .F. ) ;
#4379=AXIS2_PLACEMENT_3D ( 'NONE', #9944, #4747, #10067 ) ;
#4402=ORIENTED_EDGE ( 'NONE', *, *, #13888, .F. ) ;
#4407=ORIENTED_EDGE ( 'NONE', *, *, #14925, .T. ) ;
#4413=EDGE_CURVE ( 'NONE', #9954, #10082, #19732, .T. ) ;
#4414=DIRECTION ( 'NONE',  ( -0.4397038457472493556, 0.000000000000000000, -0.8981428216241997831 ) ) ;
#4434=VECTOR ( 'NONE', #1685, 1000.000000000000114 ) ;
#4438=CARTESIAN_POINT ( 'NONE',  ( 161.9999999999998579, 20.00000000000000000, 10.00000000000220091 ) ) ;
#4448=AXIS2_PLACEMENT_3D ( 'NONE', #9926, #20713, #4963 ) ;
#4458=AXIS2_PLACEMENT_3D ( 'NONE', #13144, #13378, #16719 ) ;
#4464=AXIS2_PLACEMENT_3D ( 'NONE', #576, #12752, #3783 ) ;
#4471=CARTESIAN_POINT ( 'NONE',  ( 161.9999999999998863, 20.00000000000000000, 8.000000000002200906 ) ) ;
#4478=ORIENTED_EDGE ( 'NONE', *, *, #15979, .T. ) ;
#4482=DIRECTION ( 'NONE',  ( 0.000000000000000000, 1.000000000000000000, -0.000000000000000000 ) ) ;
#4484=AXIS2_PLACEMENT_3D ( 'NONE', #13520, #777, #16753 ) ;
#4492=DIRECTION ( 'NONE',  ( 0.000000000000000000, 0.000000000000000000, 1.000000000000000000 ) ) ;
#4499=CIRCLE ( 'NONE', #7443, 101.0000000000000000 ) ;
#4512=DIRECTION ( 'NONE',  ( -1.000000000000000000, 0.000000000000000000, -1.362186893977296347E-14 ) ) ;
#4524=ORIENTED_EDGE ( 'NONE', *, *, #15793, .F. ) ;
#4526=CIRCLE ( 'NONE', #21026, 126.0000000000000000 ) ;
#4533=DIRECTION ( 'NONE',  ( -0.000000000000000000, -1.000000000000000000, -0.000000000000000000 ) ) ;
#4553=AXIS2_PLACEMENT_3D ( 'NONE', #17931, #19623, #12753 ) ;
#4566=ORIENTED_EDGE ( 'NONE', *, *, #8797, .F. ) ;
#4568=DIRECTION ( 'NONE',  ( 1.372099599554306628E-14, -0.000000000000000000, -1.000000000000000000 ) ) ;
#4572=ADVANCED_FACE ( 'NONE', ( #21688 ), #19857, .T. ) ;
#4573=ORIENTED_EDGE ( 'NONE', *, *, #1098, .F. ) ;
#4578=ORIENTED_EDGE ( 'NONE', *, *, #12470, .T. ) ;
#4584=DIRECTION ( 'NONE',  ( 0.000000000000000000, -1.000000000000000000, 0.000000000000000000 ) ) ;
#4596=LINE ( 'NONE', #21014, #655 ) ;
#4597=CARTESIAN_POINT ( 'NONE',  ( -158.3970384574724335, 20.00000000000000000, -62.74304228515459414 ) ) ;
#4602=DIRECTION ( 'NONE',  ( -1.396592535537253658E-14, 0.000000000000000000, -1.000000000000000000 ) ) ;
#4615=ORIENTED_EDGE ( 'NONE', *, *, #1551, .T. ) ;
#4625=CARTESIAN_POINT ( 'NONE',  ( 0.000000000000000000, 37.00000000000000711, -78.99999999999998579 ) ) ;
#4628=ORIENTED_EDGE ( 'NONE', *, *, #1917, .F. ) ;
#4630=CARTESIAN_POINT ( 'NONE',  ( 158.3970384574715808, 18.00000000000000355, 62.74304228515676130 ) ) ;
#4632=VERTEX_POINT ( 'NONE', #12881 ) ;
#4635=ADVANCED_FACE ( 'NONE', ( #6086 ), #16354, .T. ) ;
#4636=EDGE_CURVE ( 'NONE', #7423, #9056, #6573, .T. ) ;
#4641=CARTESIAN_POINT ( 'NONE',  ( 163.9999999999998579, 0.000000000000000000, 10.00000000000222933 ) ) ;
#4646=CYLINDRICAL_SURFACE ( 'NONE', #16554, 10.99999999999999289 ) ;
#4663=CYLINDRICAL_SURFACE ( 'NONE', #13750, 96.00000000000000000 ) ;
#4665=ORIENTED_EDGE ( 'NONE', *, *, #14997, .F. ) ;
#4666=DIRECTION ( 'NONE',  ( 0.000000000000000000, -1.000000000000000000, 0.000000000000000000 ) ) ;
#4669=ADVANCED_FACE ( 'NONE', ( #8029 ), #21906, .T. ) ;
#4672=EDGE_CURVE ( 'NONE', #17969, #724, #1439, .T. ) ;
#4692=CARTESIAN_POINT ( 'NONE',  ( 0.000000000000000000, 37.00000000000000711, 0.000000000000000000 ) ) ;
#4700=DIRECTION ( 'NONE',  ( -1.000000000000000000, 0.000000000000000000, 1.396592535537260757E-14 ) ) ;
#4707=ADVANCED_FACE ( 'NONE', ( #2739 ), #6297, .T. ) ;
#4721=CIRCLE ( 'NONE', #12461, 2.000000000000001776 ) ;
#4731=( BOUNDED_CURVE ( )  B_SPLINE_CURVE ( 3, ( #20272, #20728, #1558, #18996 ),
 .UNSPECIFIED., .F., .T. ) 
 B_SPLINE_CURVE_WITH_KNOTS ( ( 4, 4 ),
 ( 0.000000000000000000, 1.570796326794896558 ),
 .UNSPECIFIED. ) 
 CURVE ( )  GEOMETRIC_REPRESENTATION_ITEM ( )  RATIONAL_B_SPLINE_CURVE ( ( 1.000000000000000000, 0.8047378541243649375, 0.8047378541243649375, 1.000000000000000000 ) ) 
 REPRESENTATION_ITEM ( '' )  );
#4738=VECTOR ( 'NONE', #13774, 1000.000000000000000 ) ;
#4747=DIRECTION ( 'NONE',  ( -1.000000000000000000, 0.000000000000000000, 1.458023040593674599E-16 ) ) ;
#4760=ORIENTED_EDGE ( 'NONE', *, *, #1478, .T. ) ;
#4765=DIRECTION ( 'NONE',  ( -1.000000000000000000, 0.000000000000000000, 0.000000000000000000 ) ) ;
#4774=EDGE_CURVE ( 'NONE', #5658, #15608, #15761, .T. ) ;
#4775=ORIENTED_EDGE ( 'NONE', *, *, #4774, .T. ) ;
#4779=DIRECTION ( 'NONE',  ( 0.000000000000000000, 0.000000000000000000, -1.000000000000000000 ) ) ;
#4786=LINE ( 'NONE', #2965, #4738 ) ;
#4790=ORIENTED_EDGE ( 'NONE', *, *, #7603, .T. ) ;
#4791=CARTESIAN_POINT ( 'NONE',  ( -1.362186893977295590E-13, 20.00000000000000000, 9.999999999999994671 ) ) ;
#4801=ORIENTED_EDGE ( 'NONE', *, *, #20623, .T. ) ;
#4805=ORIENTED_EDGE ( 'NONE', *, *, #585, .F. ) ;
#4809=DIRECTION ( 'NONE',  ( 1.000000000000000000, 0.000000000000000000, -1.387778780781444413E-14 ) ) ;
#4810=DIRECTION ( 'NONE',  ( 0.4397038457472354778, 0.000000000000000000, -0.8981428216242066664 ) ) ;
#4811=DIRECTION ( 'NONE',  ( 0.000000000000000000, 0.000000000000000000, 1.000000000000000000 ) ) ;
#4813=EDGE_CURVE ( 'NONE', #8554, #18838, #3634, .T. ) ;
#4818=ORIENTED_EDGE ( 'NONE', *, *, #18267, .F. ) ;
#4846=CARTESIAN_POINT ( 'NONE',  ( -146.5000000000000000, 0.000000000000000000, 2.081668171172168513E-14 ) ) ;
#4856=CIRCLE ( 'NONE', #466, 10.00000000000000355 ) ;
#4864=DIRECTION ( 'NONE',  ( 0.000000000000000000, 0.000000000000000000, 1.000000000000000000 ) ) ;
#4866=DIRECTION ( 'NONE',  ( 1.000000000000000000, -0.000000000000000000, 1.224646799147353207E-16 ) ) ;
#4879=CARTESIAN_POINT ( 'NONE',  ( 163.9999999999992610, 18.00000000000000355, -53.76161406891485228 ) ) ;
#4880=ORIENTED_EDGE ( 'NONE', *, *, #9948, .F. ) ;
#4890=CARTESIAN_POINT ( 'NONE',  ( 0.000000000000000000, 37.00000000000000711, 0.000000000000000000 ) ) ;
#4894=ORIENTED_EDGE ( 'NONE', *, *, #11683, .F. ) ;
#4898=ADVANCED_FACE ( 'NONE', ( #6416 ), #6846, .F. ) ;
#4919=CIRCLE ( 'NONE', #17806, 2.000000000000000000 ) ;
#4933=FACE_OUTER_BOUND ( 'NONE', #5937, .T. ) ;
#4934=CARTESIAN_POINT ( 'NONE',  ( 0.000000000000000000, 0.000000000000000000, -83.99999999999998579 ) ) ;
#4935=EDGE_LOOP ( 'NONE', ( #10831, #2532, #11587, #5031 ) ) ;
#4956=DIRECTION ( 'NONE',  ( -0.000000000000000000, -1.000000000000000000, -0.000000000000000000 ) ) ;
#4963=DIRECTION ( 'NONE',  ( 0.000000000000000000, 0.000000000000000000, 1.000000000000000000 ) ) ;
#4964=ORIENTED_EDGE ( 'NONE', *, *, #20279, .T. ) ;
#4971=FACE_OUTER_BOUND ( 'NONE', #19893, .T. ) ;
#4992=AXIS2_PLACEMENT_3D ( 'NONE', #4354, #18392, #19745 ) ;
#5000=CARTESIAN_POINT ( 'NONE',  ( -146.5000000000000000, 18.00000000000000355, 10.00000000000001599 ) ) ;
#5009=CARTESIAN_POINT ( 'NONE',  ( 161.9999999999992610, 2.000000000000000000, -53.76161406891482386 ) ) ;
#5011=ADVANCED_FACE ( 'NONE', ( #7298 ), #6957, .T. ) ;
#5013=CARTESIAN_POINT ( 'NONE',  ( -164.0000000000000000, 1.999999999999998224, -53.76161406891256433 ) ) ;
#5031=ORIENTED_EDGE ( 'NONE', *, *, #13304, .F. ) ;
#5057=DIRECTION ( 'NONE',  ( 0.000000000000000000, 0.000000000000000000, -1.000000000000000000 ) ) ;
#5066=AXIS2_PLACEMENT_3D ( 'NONE', #9910, #8510, #6571 ) ;
#5068=VERTEX_POINT ( 'NONE', #11328 ) ;
#5076=EDGE_LOOP ( 'NONE', ( #10172, #6110, #1794, #4329 ) ) ;
#5080=CARTESIAN_POINT ( 'NONE',  ( -90.00000000000000000, 29.00000000000000355, -10.99999999999999289 ) ) ;
#5085=DIRECTION ( 'NONE',  ( 0.000000000000000000, 0.000000000000000000, -1.000000000000000000 ) ) ;
#5093=AXIS2_PLACEMENT_3D ( 'NONE', #14340, #21311, #9372 ) ;
#5098=ORIENTED_EDGE ( 'NONE', *, *, #11887, .T. ) ;
#5101=DIRECTION ( 'NONE',  ( 0.000000000000000000, 1.000000000000000000, 0.000000000000000000 ) ) ;
#5112=EDGE_LOOP ( 'NONE', ( #5374, #7654, #17754, #8951 ) ) ;
#5118=DIRECTION ( 'NONE',  ( 0.000000000000000000, 0.000000000000000000, 1.000000000000000000 ) ) ;
#5139=EDGE_CURVE ( 'NONE', #7464, #9403, #18680, .T. ) ;
#5142=AXIS2_PLACEMENT_3D ( 'NONE', #10381, #7256, #2096 ) ;
#5150=TOROIDAL_SURFACE ( 'NONE', #3325, 8.000000000000014211, 2.000000000000000000 ) ;
#5183=CIRCLE ( 'NONE', #4448, 8.000000000000014211 ) ;
#5190=ORIENTED_EDGE ( 'NONE', *, *, #3011, .F. ) ;
#5191=CIRCLE ( 'NONE', #827, 2.000000000000001776 ) ;
#5193=ORIENTED_EDGE ( 'NONE', *, *, #5577, .F. ) ;
#5210=CARTESIAN_POINT ( 'NONE',  ( 0.000000000000000000, 1.999999999999998224, 0.000000000000000000 ) ) ;
#5218=EDGE_LOOP ( 'NONE', ( #13370, #671, #21765, #18069 ) ) ;
#5227=ORIENTED_EDGE ( 'NONE', *, *, #19350, .T. ) ;
#5236=VERTEX_POINT ( 'NONE', #22428 ) ;
#5240=DIRECTION ( 'NONE',  ( 0.000000000000000000, 0.000000000000000000, 1.000000000000000000 ) ) ;
#5242=CIRCLE ( 'NONE', #1254, 8.000000000000003553 ) ;
#5249=AXIS2_PLACEMENT_3D ( 'NONE', #18516, #15079, #20214 ) ;
#5259=DIRECTION ( 'NONE',  ( 0.000000000000000000, 0.000000000000000000, 1.000000000000000000 ) ) ;
#5266=CARTESIAN_POINT ( 'NONE',  ( 54.52327687265659506, 1.999999999999998224, 111.3697098814018744 ) ) ;
#5272=DIRECTION ( 'NONE',  ( 0.000000000000000000, 0.000000000000000000, -1.000000000000000000 ) ) ;
#5274=ORIENTED_EDGE ( 'NONE', *, *, #17991, .F. ) ;
#5287=DIRECTION ( 'NONE',  ( -0.000000000000000000, -1.000000000000000000, -0.000000000000000000 ) ) ;
#5291=ADVANCED_FACE ( 'NONE', ( #14278 ), #14684, .T. ) ;
#5293=DIRECTION ( 'NONE',  ( -0.000000000000000000, -1.000000000000000000, -0.000000000000000000 ) ) ;
#5308=LINE ( 'NONE', #12348, #7014 ) ;
#5368=VECTOR ( 'NONE', #8036, 1000.000000000000000 ) ;
#5370=DIRECTION ( 'NONE',  ( -0.000000000000000000, -1.000000000000000000, -0.000000000000000000 ) ) ;
#5374=ORIENTED_EDGE ( 'NONE', *, *, #2751, .T. ) ;
#5378=DIRECTION ( 'NONE',  ( 0.000000000000000000, 0.000000000000000000, 1.000000000000000000 ) ) ;
#5383=ORIENTED_EDGE ( 'NONE', *, *, #6810, .F. ) ;
#5387=EDGE_CURVE ( 'NONE', #8011, #7061, #2873, .T. ) ;
#5388=ORIENTED_EDGE ( 'NONE', *, *, #669, .T. ) ;
#5414=ADVANCED_FACE ( 'NONE', ( #4252 ), #8777, .T. ) ;
#5417=ORIENTED_EDGE ( 'NONE', *, *, #15568, .F. ) ;
#5421=APPLICATION_CONTEXT ( 'automotive_design' ) ;
#5436=AXIS2_PLACEMENT_3D ( 'NONE', #1552, #8538, #13841 ) ;
#5445=ORIENTED_EDGE ( 'NONE', *, *, #16605, .T. ) ;
#5455=ORIENTED_EDGE ( 'NONE', *, *, #16572, .T. ) ;
#5468=SHAPE_REPRESENTATION ( 'Lower Angular Base Cradle Segment', ( #6292 ), #7758 ) ;
#5471=ORIENTED_EDGE ( 'NONE', *, *, #20609, .F. ) ;
#5479=CARTESIAN_POINT ( 'NONE',  ( 1.175660927181459158E-14, 0.000000000000000000, 96.00000000000000000 ) ) ;
#5487=ORIENTED_EDGE ( 'NONE', *, *, #1085, .T. ) ;
#5502=CIRCLE ( 'NONE', #9558, 8.000000000000003553 ) ;
#5505=DIRECTION ( 'NONE',  ( 0.000000000000000000, 0.000000000000000000, -1.000000000000000000 ) ) ;
#5510=EDGE_LOOP ( 'NONE', ( #11367, #9842, #10308, #515 ) ) ;
#5526=LINE ( 'NONE', #8862, #10670 ) ;
#5531=VERTEX_POINT ( 'NONE', #10903 ) ;
#5543=ORIENTED_EDGE ( 'NONE', *, *, #18624, .F. ) ;
#5553=CARTESIAN_POINT ( 'NONE',  ( 153.9999999999992610, 0.000000000000000000, -53.76161406891471017 ) ) ;
#5557=FACE_OUTER_BOUND ( 'NONE', #3485, .T. ) ;
#5577=EDGE_CURVE ( 'NONE', #5930, #19051, #14321, .T. ) ;
#5595=CLOSED_SHELL ( 'NONE', ( #12878, #13645, #14943, #6102, #6007, #15044, #17153, #12032, #21907, #21432, #6595, #3880, #15291, #8663, #13433, #2528, #19793, #7266, #15208, #17634, #12850, #8224, #13384, #15735, #4898, #13072, #12730, #4707, #14555, #18809, #21290, #2011, #2089, #7209, #6181, #2034, #6609, #13874, #4371, #8551, #16216, #16968, #9118, #16804, #4635, #11894, #1299, #18687, #14657, #5011, #17094, #15704, #1980, #3181, #20501, #4045, #5967, #5688, #16959, #11030, #11115, #3738, #5291, #20121, #19644, #9389, #13567, #17516, #16935, #4669, #21786, #7810, #11886, #1936, #5414, #16672, #2621, #21549, #3798, #22252, #4572, #12743, #12880, #7281, #9219, #12193, #12635, #19916 ) ) ;
#5598=ORIENTED_EDGE ( 'NONE', *, *, #22301, .T. ) ;
#5604=DIRECTION ( 'NONE',  ( 0.8981428216242065554, 0.000000000000000000, -0.4397038457472354223 ) ) ;
#5627=CARTESIAN_POINT ( 'NONE',  ( 0.000000000000000000, 20.00000000000000000, 0.000000000000000000 ) ) ;
#5658=VERTEX_POINT ( 'NONE', #11693 ) ;
#5663=DIRECTION ( 'NONE',  ( -0.4397038457472432493, 0.000000000000000000, -0.8981428216242028917 ) ) ;
#5665=DIRECTION ( 'NONE',  ( 1.000000000000000000, -0.000000000000000000, -1.458023040593674599E-16 ) ) ;
#5684=CARTESIAN_POINT ( 'NONE',  ( 0.000000000000000000, 18.00000000000000355, 0.000000000000000000 ) ) ;
#5688=ADVANCED_FACE ( 'NONE', ( #2846 ), #16877, .T. ) ;
#5701=CARTESIAN_POINT ( 'NONE',  ( -164.0000000000000000, 18.00000000000000355, 8.000000000000019540 ) ) ;
#5720=CARTESIAN_POINT ( 'NONE',  ( -164.0000000000000284, 0.8284271247461896248, -7.999999999999978684 ) ) ;
#5721=DIRECTION ( 'NONE',  ( 0.000000000000000000, 0.000000000000000000, 1.000000000000000000 ) ) ;
#5729=DIRECTION ( 'NONE',  ( 0.000000000000000000, 1.000000000000000000, -0.000000000000000000 ) ) ;
#5746=CARTESIAN_POINT ( 'NONE',  ( -163.1715728752537871, 20.00000000000000000, 8.828427124746209387 ) ) ;
#5756=CARTESIAN_POINT ( 'NONE',  ( -146.5000000000000000, 0.000000000000000000, 10.00000000000001599 ) ) ;
#5769=DIRECTION ( 'NONE',  ( -0.000000000000000000, -1.000000000000000000, -0.000000000000000000 ) ) ;
#5773=DIRECTION ( 'NONE',  ( 0.8981428216242086648, -0.000000000000000000, 0.4397038457472312589 ) ) ;
#5776=VECTOR ( 'NONE', #10122, 1000.000000000000114 ) ;
#5780=DIRECTION ( 'NONE',  ( 0.4397038457472354778, 0.000000000000000000, -0.8981428216242066664 ) ) ;
#5791=CARTESIAN_POINT ( 'NONE',  ( 163.9999999999998863, 1.999999999999998224, -8.000000000002268408 ) ) ;
#5806=DIRECTION ( 'NONE',  ( -0.8981428216242027807, -0.000000000000000000, 0.4397038457472431938 ) ) ;
#5807=CARTESIAN_POINT ( 'NONE',  ( -101.0000000000000000, 37.00000000000000711, 0.000000000000000000 ) ) ;
#5810=ORIENTED_EDGE ( 'NONE', *, *, #4636, .F. ) ;
#5827=CARTESIAN_POINT ( 'NONE',  ( -157.5176307659779127, 18.00000000000000355, 60.94675664190624786 ) ) ;
#5844=FACE_OUTER_BOUND ( 'NONE', #8233, .T. ) ;
#5849=DIRECTION ( 'NONE',  ( 0.8981428216242089979, 0.000000000000000000, 0.4397038457472307593 ) ) ;
#5867=DIRECTION ( 'NONE',  ( 1.387778780781444571E-14, 0.000000000000000000, -1.000000000000000000 ) ) ;
#5870=DIRECTION ( 'NONE',  ( 0.000000000000000000, 0.000000000000000000, 1.000000000000000000 ) ) ;
#5873=DIRECTION ( 'NONE',  ( 0.000000000000000000, 1.000000000000000000, 0.000000000000000000 ) ) ;
#5876=DIRECTION ( 'NONE',  ( 0.000000000000000000, 1.000000000000000000, -0.000000000000000000 ) ) ;
#5881=CIRCLE ( 'NONE', #16557, 118.0000000000000000 ) ;
#5895=FACE_BOUND ( 'NONE', #14585, .T. ) ;
#5900=DIRECTION ( 'NONE',  ( -0.4397038457472424167, 0.000000000000000000, -0.8981428216242032248 ) ) ;
#5908=DIRECTION ( 'NONE',  ( 0.000000000000000000, 1.000000000000000000, -0.000000000000000000 ) ) ;
#5918=AXIS2_PLACEMENT_3D ( 'NONE', #16588, #4257, #9428 ) ;
#5922=EDGE_LOOP ( 'NONE', ( #22372, #13643, #5471, #9555 ) ) ;
#5925=CARTESIAN_POINT ( 'NONE',  ( -54.52327687265814404, 1.999999999999998224, 111.3697098814011923 ) ) ;
#5930=VERTEX_POINT ( 'NONE', #1926 ) ;
#5937=EDGE_LOOP ( 'NONE', ( #16453, #18875, #9271, #15919 ) ) ;
#5944=VECTOR ( 'NONE', #6862, 1000.000000000000227 ) ;
#5945=AXIS2_PLACEMENT_3D ( 'NONE', #9487, #12964, #775 ) ;
#5946=DIRECTION ( 'NONE',  ( 1.776356839400250465E-15, 0.000000000000000000, 1.000000000000000000 ) ) ;
#5963=AXIS2_PLACEMENT_3D ( 'NONE', #5000, #14221, #77 ) ;
#5964=AXIS2_PLACEMENT_3D ( 'NONE', #16591, #21812, #6103 ) ;
#5967=ADVANCED_FACE ( 'NONE', ( #20276 ), #18334, .T. ) ;
#5968=CYLINDRICAL_SURFACE ( 'NONE', #1806, 126.0000000000000000 ) ;
#5986=ORIENTED_EDGE ( 'NONE', *, *, #7817, .T. ) ;
#5992=CARTESIAN_POINT ( 'NONE',  ( 0.000000000000000000, 20.00000000000000000, 0.000000000000000000 ) ) ;
#5996=TOROIDAL_SURFACE ( 'NONE', #18828, 8.000000000000014211, 2.000000000000000000 ) ;
#6007=ADVANCED_FACE ( 'NONE', ( #13748 ), #13417, .T. ) ;
#6017=LINE ( 'NONE', #11417, #8917 ) ;
#6024=ORIENTED_EDGE ( 'NONE', *, *, #6810, .T. ) ;
#6030=DIRECTION ( 'NONE',  ( -0.000000000000000000, -1.000000000000000000, -0.000000000000000000 ) ) ;
#6057=CARTESIAN_POINT ( 'NONE',  ( -7.930164461608248607E-16, 20.00000000000000000, -7.999999999999994671 ) ) ;
#6070=EDGE_LOOP ( 'NONE', ( #7754, #21406, #1972, #15939 ) ) ;
#6072=CARTESIAN_POINT ( 'NONE',  ( -101.0000000000000000, 29.00000000000000355, 0.000000000000000000 ) ) ;
#6086=FACE_OUTER_BOUND ( 'NONE', #12984, .T. ) ;
#6095=ORIENTED_EDGE ( 'NONE', *, *, #19326, .F. ) ;
#6100=CARTESIAN_POINT ( 'NONE',  ( 0.000000000000000000, 1.999999999999998224, 0.000000000000000000 ) ) ;
#6101=PLANE ( 'NONE',  #5918 ) ;
#6102=ADVANCED_FACE ( 'NONE', ( #20385 ), #4646, .F. ) ;
#6103=DIRECTION ( 'NONE',  ( 1.386679829960243061E-14, 0.000000000000000000, 1.000000000000000000 ) ) ;
#6110=ORIENTED_EDGE ( 'NONE', *, *, #13658, .F. ) ;
#6119=CYLINDRICAL_SURFACE ( 'NONE', #4458, 10.00000000000000888 ) ;
#6120=CARTESIAN_POINT ( 'NONE',  ( -90.00000000000000000, 45.00100000000000477, -10.99999999999999289 ) ) ;
#6125=ORIENTED_EDGE ( 'NONE', *, *, #21705, .F. ) ;
#6131=EDGE_CURVE ( 'NONE', #3408, #14037, #8891, .T. ) ;
#6132=CARTESIAN_POINT ( 'NONE',  ( 146.4999999999998579, 20.00000000000000000, 9.999999999997978506 ) ) ;
#6137=CARTESIAN_POINT ( 'NONE',  ( 55.40268456415105902, 18.00000000000000355, -113.1659955246503699 ) ) ;
#6142=CARTESIAN_POINT ( 'NONE',  ( -162.0000000000000000, 0.000000000000000000, 8.000000000000019540 ) ) ;
#6153=ORIENTED_EDGE ( 'NONE', *, *, #9991, .F. ) ;
#6172=AXIS2_PLACEMENT_3D ( 'NONE', #643, #16634, #11100 ) ;
#6174=DIRECTION ( 'NONE',  ( -0.000000000000000000, -1.000000000000000000, -0.000000000000000000 ) ) ;
#6181=ADVANCED_FACE ( 'NONE', ( #5557 ), #12589, .F. ) ;
#6183=ORIENTED_EDGE ( 'NONE', *, *, #9948, .T. ) ;
#6192=AXIS2_PLACEMENT_3D ( 'NONE', #22021, #6326, #13345 ) ;
#6195=EDGE_CURVE ( 'NONE', #18453, #4632, #14999, .T. ) ;
#6203=DIRECTION ( 'NONE',  ( 0.000000000000000000, 1.000000000000000000, -0.000000000000000000 ) ) ;
#6233=DIRECTION ( 'NONE',  ( -0.000000000000000000, -1.000000000000000000, -0.000000000000000000 ) ) ;
#6234=LINE ( 'NONE', #6120, #22302 ) ;
#6241=ORIENTED_EDGE ( 'NONE', *, *, #14703, .T. ) ;
#6252=VERTEX_POINT ( 'NONE', #7521 ) ;
#6254=FACE_OUTER_BOUND ( 'NONE', #14047, .T. ) ;
#6260=VERTEX_POINT ( 'NONE', #2461 ) ;
#6261=EDGE_CURVE ( 'NONE', #9056, #21621, #15457, .T. ) ;
#6278=EDGE_CURVE ( 'NONE', #19256, #17288, #12125, .T. ) ;
#6280=AXIS2_PLACEMENT_3D ( 'NONE', #16623, #21736, #874 ) ;
#6292=AXIS2_PLACEMENT_3D ( 'NONE', #3102, #12069, #1395 ) ;
#6297=CYLINDRICAL_SURFACE ( 'NONE', #2156, 126.0000000000000000 ) ;
#6326=DIRECTION ( 'NONE',  ( -0.000000000000000000, -1.000000000000000000, -0.000000000000000000 ) ) ;
#6348=EDGE_CURVE ( 'NONE', #7061, #4119, #11399, .T. ) ;
#6359=DIRECTION ( 'NONE',  ( -1.000000000000000000, 0.000000000000000000, -1.362186893977296347E-14 ) ) ;
#6363=CARTESIAN_POINT ( 'NONE',  ( 161.9999999999992610, 20.00000000000000000, 53.76161406891478123 ) ) ;
#6364=VERTEX_POINT ( 'NONE', #6132 ) ;
#6391=DIRECTION ( 'NONE',  ( -0.000000000000000000, -1.000000000000000000, -0.000000000000000000 ) ) ;
#6399=CARTESIAN_POINT ( 'NONE',  ( -55.40268456415264353, 20.00000000000000000, -113.1659955246495883 ) ) ;
#6400=AXIS2_PLACEMENT_3D ( 'NONE', #22037, #10007, #4810 ) ;
#6402=EDGE_LOOP ( 'NONE', ( #8469, #19215, #12209, #359 ) ) ;
#6407=EDGE_LOOP ( 'NONE', ( #5098, #19621, #11532, #1873 ) ) ;
#6416=FACE_OUTER_BOUND ( 'NONE', #8783, .T. ) ;
#6427=EDGE_CURVE ( 'NONE', #3659, #22165, #9181, .T. ) ;
#6433=EDGE_CURVE ( 'NONE', #1407, #2837, #5526, .T. ) ;
#6439=ORIENTED_EDGE ( 'NONE', *, *, #6278, .T. ) ;
#6462=ORIENTED_EDGE ( 'NONE', *, *, #11910, .F. ) ;
#6474=DIRECTION ( 'NONE',  ( 0.000000000000000000, 0.000000000000000000, 1.000000000000000000 ) ) ;
#6478=DIRECTION ( 'NONE',  ( 0.000000000000000000, -1.000000000000000000, 0.000000000000000000 ) ) ;
#6489=ORIENTED_EDGE ( 'NONE', *, *, #1241, .F. ) ;
#6496=EDGE_CURVE ( 'NONE', #7803, #7424, #6635, .T. ) ;
#6498=CARTESIAN_POINT ( 'NONE',  ( -157.5176307659779411, 18.00000000000000355, -60.94675664190618392 ) ) ;
#6505=CARTESIAN_POINT ( 'NONE',  ( -146.5000000000000000, 20.00000000000000000, 2.081668171172168513E-14 ) ) ;
#6509=LINE ( 'NONE', #13524, #4434 ) ;
#6537=EDGE_LOOP ( 'NONE', ( #21168, #13651, #7264, #7528 ) ) ;
#6543=DIRECTION ( 'NONE',  ( 0.000000000000000000, 1.000000000000000000, -0.000000000000000000 ) ) ;
#6545=AXIS2_PLACEMENT_3D ( 'NONE', #10732, #10849, #14198 ) ;
#6554=EDGE_LOOP ( 'NONE', ( #19637, #21634, #4407, #16604 ) ) ;
#6564=ORIENTED_EDGE ( 'NONE', *, *, #16572, .F. ) ;
#6571=DIRECTION ( 'NONE',  ( 0.000000000000000000, 0.000000000000000000, 1.000000000000000000 ) ) ;
#6573=CIRCLE ( 'NONE', #9506, 126.0000000000000000 ) ;
#6576=VERTEX_POINT ( 'NONE', #2961 ) ;
#6591=AXIS2_PLACEMENT_3D ( 'NONE', #1640, #15440, #5057 ) ;
#6595=ADVANCED_FACE ( 'NONE', ( #13030 ), #15174, .T. ) ;
#6609=ADVANCED_FACE ( 'NONE', ( #22126, #14524 ), #19876, .T. ) ;
#6612=DIRECTION ( 'NONE',  ( 0.000000000000000000, 0.000000000000000000, -1.000000000000000000 ) ) ;
#6620=FACE_OUTER_BOUND ( 'NONE', #14710, .T. ) ;
#6622=( BOUNDED_CURVE ( )  B_SPLINE_CURVE ( 3, ( #12489, #14567, #7541, #540 ),
 .UNSPECIFIED., .F., .T. ) 
 B_SPLINE_CURVE_WITH_KNOTS ( ( 4, 4 ),
 ( 3.141592653589793560, 4.712388980384689674 ),
 .UNSPECIFIED. ) 
 CURVE ( )  GEOMETRIC_REPRESENTATION_ITEM ( )  RATIONAL_B_SPLINE_CURVE ( ( 1.000000000000000000, 0.8047378541243650485, 0.8047378541243650485, 1.000000000000000000 ) ) 
 REPRESENTATION_ITEM ( '' )  );
#6630=EDGE_LOOP ( 'NONE', ( #2272, #246, #7193, #13783 ) ) ;
#6635=CIRCLE ( 'NONE', #5142, 120.0000000000000000 ) ;
#6650=EDGE_CURVE ( 'NONE', #11917, #168, #20561, .T. ) ;
#6671=FACE_OUTER_BOUND ( 'NONE', #22443, .T. ) ;
#6675=CIRCLE ( 'NONE', #12540, 10.00000000000000888 ) ;
#6687=FACE_OUTER_BOUND ( 'NONE', #17438, .T. ) ;
#6689=VECTOR ( 'NONE', #21629, 1000.000000000000000 ) ;
#6702=VECTOR ( 'NONE', #3653, 1000.000000000000114 ) ;
#6706=ORIENTED_EDGE ( 'NONE', *, *, #21573, .F. ) ;
#6711=EDGE_LOOP ( 'NONE', ( #16225, #19008, #15681, #7851 ) ) ;
#6722=CARTESIAN_POINT ( 'NONE',  ( 146.4999999999998863, 20.00000000000000000, -8.000000000002026823 ) ) ;
#6747=AXIS2_PLACEMENT_3D ( 'NONE', #13294, #4533, #11905 ) ;
#6754=CIRCLE ( 'NONE', #2382, 110.1134477342067157 ) ;
#6761=EDGE_LOOP ( 'NONE', ( #5986, #5388, #6778, #20852 ) ) ;
#6767=ORIENTED_EDGE ( 'NONE', *, *, #12375, .F. ) ;
#6778=ORIENTED_EDGE ( 'NONE', *, *, #10918, .F. ) ;
#6791=DIRECTION ( 'NONE',  ( -0.000000000000000000, -1.000000000000000000, -0.000000000000000000 ) ) ;
#6802=DIRECTION ( 'NONE',  ( 1.387778780781445676E-14, 0.000000000000000000, -1.000000000000000000 ) ) ;
#6810=EDGE_CURVE ( 'NONE', #7475, #2837, #13295, .T. ) ;
#6814=ORIENTED_EDGE ( 'NONE', *, *, #15793, .T. ) ;
#6815=ORIENTED_EDGE ( 'NONE', *, *, #16561, .T. ) ;
#6818=EDGE_LOOP ( 'NONE', ( #2426, #14125, #5383, #14158 ) ) ;
#6819=DIRECTION ( 'NONE',  ( 1.362186893977296347E-14, 0.000000000000000000, -1.000000000000000000 ) ) ;
#6839=CIRCLE ( 'NONE', #4992, 78.99999999999998579 ) ;
#6846=PLANE ( 'NONE',  #2917 ) ;
#6856=CARTESIAN_POINT ( 'NONE',  ( 163.9999999999998295, 19.17157287525381193, 8.000000000002229328 ) ) ;
#6862=DIRECTION ( 'NONE',  ( 0.000000000000000000, -0.9455185755993167351, 0.3255681544571568109 ) ) ;
#6864=CARTESIAN_POINT ( 'NONE',  ( 1.236893267138826732E-14, 29.00000000000000355, 101.0000000000000000 ) ) ;
#6865=ORIENTED_EDGE ( 'NONE', *, *, #10366, .T. ) ;
#6872=ORIENTED_EDGE ( 'NONE', *, *, #155, .F. ) ;
#6874=CARTESIAN_POINT ( 'NONE',  ( 146.5000000000000000, 1.999999999999998224, -2.025191382850354537E-12 ) ) ;
#6885=CARTESIAN_POINT ( 'NONE',  ( -54.52327687265815825, 18.00000000000000355, -111.3697098814011923 ) ) ;
#6908=EDGE_LOOP ( 'NONE', ( #10585, #22520, #10678, #3911 ) ) ;
#6917=CARTESIAN_POINT ( 'NONE',  ( 0.000000000000000000, 37.00000000000000711, -83.99999999999998579 ) ) ;
#6919=CARTESIAN_POINT ( 'NONE',  ( 0.000000000000000000, 29.00000000000000355, 0.000000000000000000 ) ) ;
#6922=FACE_OUTER_BOUND ( 'NONE', #17862, .T. ) ;
#6925=CARTESIAN_POINT ( 'NONE',  ( -9.912705577010312730E-16, 1.999999999999998224, -9.999999999999994671 ) ) ;
#6926=VECTOR ( 'NONE', #13550, 1000.000000000000000 ) ;
#6937=AXIS2_PLACEMENT_3D ( 'NONE', #8320, #10586, #12435 ) ;
#6944=EDGE_CURVE ( 'NONE', #20064, #10751, #13276, .T. ) ;
#6954=EDGE_CURVE ( 'NONE', #2665, #15942, #16227, .T. ) ;
#6957=CYLINDRICAL_SURFACE ( 'NONE', #5093, 2.000000000000001776 ) ;
#6977=EDGE_CURVE ( 'NONE', #4119, #8602, #16315, .T. ) ;
#6994=CIRCLE ( 'NONE', #12156, 10.99999999999999289 ) ;
#7002=DIRECTION ( 'NONE',  ( -0.4397038457472354778, 0.000000000000000000, -0.8981428216242066664 ) ) ;
#7014=VECTOR ( 'NONE', #21165, 1000.000000000000000 ) ;
#7037=ORIENTED_EDGE ( 'NONE', *, *, #11529, .F. ) ;
#7044=ORIENTED_EDGE ( 'NONE', *, *, #17432, .T. ) ;
#7050=DIRECTION ( 'NONE',  ( -9.912705577010319386E-17, 0.000000000000000000, -1.000000000000000000 ) ) ;
#7061=VERTEX_POINT ( 'NONE', #11232 ) ;
#7068=ORIENTED_EDGE ( 'NONE', *, *, #19159, .F. ) ;
#7075=AXIS2_PLACEMENT_3D ( 'NONE', #2130, #15713, #17544 ) ;
#7082=LINE ( 'NONE', #10766, #16684 ) ;
#7100=DIRECTION ( 'NONE',  ( 0.000000000000000000, 0.000000000000000000, 1.000000000000000000 ) ) ;
#7105=CARTESIAN_POINT ( 'NONE',  ( -162.0000000000000000, 20.00000000000000000, 53.76161406891260697 ) ) ;
#7111=DIRECTION ( 'NONE',  ( 0.000000000000000000, 0.000000000000000000, 1.000000000000000000 ) ) ;
#7160=CIRCLE ( 'NONE', #15271, 101.0000000000000000 ) ;
#7170=DIRECTION ( 'NONE',  ( 1.396592535537253658E-14, 0.000000000000000000, 1.000000000000000000 ) ) ;
#7174=AXIS2_PLACEMENT_3D ( 'NONE', #22253, #6543, #7111 ) ;
#7182=ORIENTED_EDGE ( 'NONE', *, *, #9835, .F. ) ;
#7187=AXIS2_PLACEMENT_3D ( 'NONE', #20775, #10451, #1721 ) ;
#7193=ORIENTED_EDGE ( 'NONE', *, *, #9657, .F. ) ;
#7209=ADVANCED_FACE ( 'NONE', ( #16484 ), #6119, .T. ) ;
#7231=FACE_OUTER_BOUND ( 'NONE', #5510, .T. ) ;
#7239=ORIENTED_EDGE ( 'NONE', *, *, #4672, .F. ) ;
#7253=CARTESIAN_POINT ( 'NONE',  ( 0.000000000000000000, 1.999999999999998224, 0.000000000000000000 ) ) ;
#7256=DIRECTION ( 'NONE',  ( 0.000000000000000000, 1.000000000000000000, 0.000000000000000000 ) ) ;
#7262=DIRECTION ( 'NONE',  ( 0.000000000000000000, 0.000000000000000000, -1.000000000000000000 ) ) ;
#7263=EDGE_LOOP ( 'NONE', ( #1440, #22595, #22106, #18815 ) ) ;
#7264=ORIENTED_EDGE ( 'NONE', *, *, #9282, .F. ) ;
#7266=ADVANCED_FACE ( 'NONE', ( #2690 ), #9695, .T. ) ;
#7273=AXIS2_PLACEMENT_3D ( 'NONE', #20258, #6030, #2812 ) ;
#7274=DIRECTION ( 'NONE',  ( -1.000000000000000000, 0.000000000000000000, 1.396592535537253658E-14 ) ) ;
#7277=DIRECTION ( 'NONE',  ( 0.000000000000000000, 0.000000000000000000, 1.000000000000000000 ) ) ;
#7281=ADVANCED_FACE ( 'NONE', ( #16817 ), #1071, .T. ) ;
#7298=FACE_OUTER_BOUND ( 'NONE', #6407, .T. ) ;
#7355=DIRECTION ( 'NONE',  ( -0.000000000000000000, -1.000000000000000000, 0.000000000000000000 ) ) ;
#7362=CARTESIAN_POINT ( 'NONE',  ( 0.000000000000000000, 20.00000000000000000, 124.0000000000000000 ) ) ;
#7371=CYLINDRICAL_SURFACE ( 'NONE', #14358, 10.00000000000001599 ) ;
#7375=ORIENTED_EDGE ( 'NONE', *, *, #17938, .F. ) ;
#7377=VERTEX_POINT ( 'NONE', #20571 ) ;
#7382=ORIENTED_EDGE ( 'NONE', *, *, #2951, .F. ) ;
#7389=CIRCLE ( 'NONE', #17309, 8.000000000000014211 ) ;
#7392=DIRECTION ( 'NONE',  ( -0.000000000000000000, -1.000000000000000000, 0.000000000000000000 ) ) ;
#7393=DIRECTION ( 'NONE',  ( 0.000000000000000000, 1.000000000000000000, -0.000000000000000000 ) ) ;
#7394=VECTOR ( 'NONE', #18935, 1000.000000000000114 ) ;
#7412=TOROIDAL_SURFACE ( 'NONE', #15148, 124.0000000000000000, 2.000000000000000000 ) ;
#7421=ORIENTED_EDGE ( 'NONE', *, *, #19002, .T. ) ;
#7423=VERTEX_POINT ( 'NONE', #22605 ) ;
#7424=VERTEX_POINT ( 'NONE', #15661 ) ;
#7426=CARTESIAN_POINT ( 'NONE',  ( 163.9999999999992610, 20.00000000000000000, 53.76161406891480965 ) ) ;
#7433=DIRECTION ( 'NONE',  ( -1.000000000000000000, 0.000000000000000000, -1.387778780781444413E-14 ) ) ;
#7435=DIRECTION ( 'NONE',  ( 0.000000000000000000, 0.000000000000000000, -1.000000000000000000 ) ) ;
#7438=VERTEX_POINT ( 'NONE', #10245 ) ;
#7443=AXIS2_PLACEMENT_3D ( 'NONE', #4890, #16062, #2028 ) ;
#7445=EDGE_CURVE ( 'NONE', #10110, #10707, #17145, .T. ) ;
#7450=ADVANCED_BREP_SHAPE_REPRESENTATION ( '', ( #9845, #6292 ), #7758 ) ;
#7459=PLANE ( 'NONE',  #4553 ) ;
#7463=CIRCLE ( 'NONE', #11127, 2.000000000000007550 ) ;
#7464=VERTEX_POINT ( 'NONE', #13921 ) ;
#7466=CARTESIAN_POINT ( 'NONE',  ( -162.0000000000000000, 0.000000000000000000, 10.00000000000001776 ) ) ;
#7469=DIRECTION ( 'NONE',  ( -0.000000000000000000, -1.000000000000000000, -0.000000000000000000 ) ) ;
#7473=VECTOR ( 'NONE', #15809, 1000.000000000000114 ) ;
#7475=VERTEX_POINT ( 'NONE', #15775 ) ;
#7476=CONICAL_SURFACE ( 'NONE', #6747, 117.0000000000000000, 0.3316125578789227979 ) ;
#7503=ORIENTED_EDGE ( 'NONE', *, *, #6131, .T. ) ;
#7515=FACE_OUTER_BOUND ( 'NONE', #21381, .T. ) ;
#7521=CARTESIAN_POINT ( 'NONE',  ( -164.0000000000000000, 18.00000000000000355, -7.999999999999979572 ) ) ;
#7528=ORIENTED_EDGE ( 'NONE', *, *, #14135, .F. ) ;
#7536=CARTESIAN_POINT ( 'NONE',  ( 146.4999999999998579, 0.000000000000000000, -10.00000000000202682 ) ) ;
#7537=CARTESIAN_POINT ( 'NONE',  ( 163.9999999999998863, 1.999999999999998224, 8.000000000002229328 ) ) ;
#7541=CARTESIAN_POINT ( 'NONE',  ( 163.1715728752537018, -2.184664232470859687E-16, 8.828427124748404964 ) ) ;
#7558=ORIENTED_EDGE ( 'NONE', *, *, #19238, .T. ) ;
#7564=CARTESIAN_POINT ( 'NONE',  ( -154.0000000000000000, 18.00000000000000355, 53.76161406891259986 ) ) ;
#7572=VERTEX_POINT ( 'NONE', #12769 ) ;
#7578=CARTESIAN_POINT ( 'NONE',  ( -164.0000000000000284, 0.8284271247461896248, 8.000000000000019540 ) ) ;
#7584=CARTESIAN_POINT ( 'NONE',  ( 0.000000000000000000, 0.000000000000000000, 0.000000000000000000 ) ) ;
#7603=EDGE_CURVE ( 'NONE', #7438, #22518, #5191, .T. ) ;
#7654=ORIENTED_EDGE ( 'NONE', *, *, #16525, .F. ) ;
#7678=LINE ( 'NONE', #14719, #14773 ) ;
#7688=ORIENTED_EDGE ( 'NONE', *, *, #9835, .T. ) ;
#7694=DIRECTION ( 'NONE',  ( 0.000000000000000000, 0.000000000000000000, -1.000000000000000000 ) ) ;
#7703=AXIS2_PLACEMENT_3D ( 'NONE', #16490, #9582, #2456 ) ;
#7744=AXIS2_PLACEMENT_3D ( 'NONE', #20308, #607, #5870 ) ;
#7746=DIRECTION ( 'NONE',  ( 1.387778780781445676E-14, 0.000000000000000000, 1.000000000000000000 ) ) ;
#7754=ORIENTED_EDGE ( 'NONE', *, *, #17676, .T. ) ;
#7758=( GEOMETRIC_REPRESENTATION_CONTEXT ( 3 ) GLOBAL_UNCERTAINTY_ASSIGNED_CONTEXT ( ( #13837 ) ) GLOBAL_UNIT_ASSIGNED_CONTEXT ( ( #17274, #11652, #3135 ) ) REPRESENTATION_CONTEXT ( 'NONE', 'WORKASPACE' ) );
#7760=CARTESIAN_POINT ( 'NONE',  ( 0.000000000000000000, 37.00000000000000711, 0.000000000000000000 ) ) ;
#7761=AXIS2_PLACEMENT_3D ( 'NONE', #11746, #3349, #13587 ) ;
#7779=VERTEX_POINT ( 'NONE', #18278 ) ;
#7793=ORIENTED_EDGE ( 'NONE', *, *, #11607, .F. ) ;
#7799=CARTESIAN_POINT ( 'NONE',  ( 55.40268456415110165, 1.999999999999998224, 113.1659955246503415 ) ) ;
#7800=CARTESIAN_POINT ( 'NONE',  ( -163.1715728752537871, -6.488953147413177264E-16, -8.828427124746170307 ) ) ;
#7803=VERTEX_POINT ( 'NONE', #11378 ) ;
#7810=ADVANCED_FACE ( 'NONE', ( #2658 ), #11844, .T. ) ;
#7812=CARTESIAN_POINT ( 'NONE',  ( -55.40268456415261511, 1.999999999999998224, 113.1659955246496025 ) ) ;
#7815=EDGE_CURVE ( 'NONE', #20064, #15219, #20204, .T. ) ;
#7817=EDGE_CURVE ( 'NONE', #3254, #4632, #18506, .T. ) ;
#7820=DIRECTION ( 'NONE',  ( 0.000000000000000000, 0.000000000000000000, 1.000000000000000000 ) ) ;
#7838=( NAMED_UNIT ( * ) PLANE_ANGLE_UNIT ( ) SI_UNIT ( $, .RADIAN. ) );
#7840=CARTESIAN_POINT ( 'NONE',  ( -154.0000000000000000, 1.999999999999998224, -53.76161406891256433 ) ) ;
#7844=ORIENTED_EDGE ( 'NONE', *, *, #4413, .T. ) ;
#7846=VERTEX_POINT ( 'NONE', #21002 ) ;
#7848=AXIS2_PLACEMENT_3D ( 'NONE', #3495, #8540, #10852 ) ;
#7851=ORIENTED_EDGE ( 'NONE', *, *, #17991, .T. ) ;
#7874=ORIENTED_EDGE ( 'NONE', *, *, #19748, .F. ) ;
#7906=VERTEX_POINT ( 'NONE', #18710 ) ;
#7913=CARTESIAN_POINT ( 'NONE',  ( 158.3970384574715524, 18.00000000000000355, -62.74304228515679682 ) ) ;
#7919=CARTESIAN_POINT ( 'NONE',  ( -146.5000000000000000, 18.00000000000000355, 8.000000000000017764 ) ) ;
#7923=DIRECTION ( 'NONE',  ( -0.000000000000000000, -1.000000000000000000, 0.000000000000000000 ) ) ;
#7927=DIRECTION ( 'NONE',  ( -1.000000000000000000, 0.000000000000000000, 9.912705577010318154E-17 ) ) ;
#7939=FACE_OUTER_BOUND ( 'NONE', #10560, .T. ) ;
#7942=EDGE_CURVE ( 'NONE', #6252, #11917, #20771, .T. ) ;
#7949=ORIENTED_EDGE ( 'NONE', *, *, #561, .F. ) ;
#7958=CARTESIAN_POINT ( 'NONE',  ( 3.086109933851330151E-14, 20.00000000000000000, 126.0000000000000000 ) ) ;
#7977=DIRECTION ( 'NONE',  ( 0.8981428216241984508, 0.000000000000000000, -0.4397038457472520756 ) ) ;
#7993=VERTEX_POINT ( 'NONE', #10449 ) ;
#8005=PLANE ( 'NONE',  #18812 ) ;
#8007=AXIS2_PLACEMENT_3D ( 'NONE', #9782, #16795, #1047 ) ;
#8008=VERTEX_POINT ( 'NONE', #21117 ) ;
#8011=VERTEX_POINT ( 'NONE', #12301 ) ;
#8022=ORIENTED_EDGE ( 'NONE', *, *, #14210, .T. ) ;
#8026=VECTOR ( 'NONE', #15514, 1000.000000000000114 ) ;
#8029=FACE_OUTER_BOUND ( 'NONE', #8591, .T. ) ;
#8036=DIRECTION ( 'NONE',  ( 1.000000000000000000, -0.000000000000000000, -1.386679829960243376E-14 ) ) ;
#8044=DIRECTION ( 'NONE',  ( -0.8981428216242027807, 0.000000000000000000, 0.4397038457472431938 ) ) ;
#8046=CARTESIAN_POINT ( 'NONE',  ( 1.166418432474939088E-15, 20.00000000000000000, 7.999999999999994671 ) ) ;
#8049=ORIENTED_EDGE ( 'NONE', *, *, #12333, .T. ) ;
#8051=DIRECTION ( 'NONE',  ( -0.000000000000000000, -1.000000000000000000, -0.000000000000000000 ) ) ;
#8076=DIRECTION ( 'NONE',  ( 0.000000000000000000, 0.000000000000000000, -1.000000000000000000 ) ) ;
#8118=ORIENTED_EDGE ( 'NONE', *, *, #18410, .T. ) ;
#8137=CARTESIAN_POINT ( 'NONE',  ( 54.52327687265660927, 1.999999999999998224, -111.3697098814019313 ) ) ;
#8140=DIRECTION ( 'NONE',  ( 0.000000000000000000, 0.000000000000000000, -1.000000000000000000 ) ) ;
#8153=AXIS2_PLACEMENT_3D ( 'NONE', #6072, #2514, #918 ) ;
#8166=DIRECTION ( 'NONE',  ( -0.000000000000000000, -1.000000000000000000, -0.000000000000000000 ) ) ;
#8169=LINE ( 'NONE', #10121, #2726 ) ;
#8172=AXIS2_PLACEMENT_3D ( 'NONE', #8248, #20513, #17317 ) ;
#8187=CIRCLE ( 'NONE', #20632, 10.00000000000000888 ) ;
#8190=ORIENTED_EDGE ( 'NONE', *, *, #10736, .F. ) ;
#8191=TOROIDAL_SURFACE ( 'NONE', #3789, 8.000000000000014211, 2.000000000000000000 ) ;
#8192=CYLINDRICAL_SURFACE ( 'NONE', #7761, 120.0000000000000000 ) ;
#8195=CARTESIAN_POINT ( 'NONE',  ( 146.4999999999998863, 1.999999999999998224, -8.000000000002026823 ) ) ;
#8208=AXIS2_PLACEMENT_3D ( 'NONE', #10735, #1774, #5085 ) ;
#8210=CARTESIAN_POINT ( 'NONE',  ( 162.0000000000000000, 18.00000000000000355, -2.262479907570351121E-12 ) ) ;
#8211=LINE ( 'NONE', #11996, #16595 ) ;
#8222=CIRCLE ( 'NONE', #4175, 126.0000000000000000 ) ;
#8224=ADVANCED_FACE ( 'NONE', ( #1014 ), #8005, .T. ) ;
#8227=LINE ( 'NONE', #6722, #10037 ) ;
#8233=EDGE_LOOP ( 'NONE', ( #4665, #19244, #4615, #20842 ) ) ;
#8248=CARTESIAN_POINT ( 'NONE',  ( -154.0000000000000000, 1.999999999999998224, -53.76161406891256433 ) ) ;
#8250=EDGE_LOOP ( 'NONE', ( #12062, #19828 ) ) ;
#8254=DIRECTION ( 'NONE',  ( -0.000000000000000000, -1.000000000000000000, -0.000000000000000000 ) ) ;
#8257=DIRECTION ( 'NONE',  ( 0.000000000000000000, 1.000000000000000000, 0.000000000000000000 ) ) ;
#8269=CARTESIAN_POINT ( 'NONE',  ( 0.000000000000000000, 25.00000000000000000, 0.000000000000000000 ) ) ;
#8271=MECHANICAL_DESIGN_GEOMETRIC_PRESENTATION_REPRESENTATION('',(#1309),#21459);
#8273=DIRECTION ( 'NONE',  ( 1.000000000000000000, -0.000000000000000000, -1.386679829960243376E-14 ) ) ;
#8278=CARTESIAN_POINT ( 'NONE',  ( -154.0000000000000000, 0.000000000000000000, -53.76161406891256433 ) ) ;
#8282=CARTESIAN_POINT ( 'NONE',  ( 162.0000000000000000, 18.00000000000000355, 2.222801351277976832E-12 ) ) ;
#8292=VERTEX_POINT ( 'NONE', #22562 ) ;
#8320=CARTESIAN_POINT ( 'NONE',  ( -146.5000000000000000, 18.00000000000000355, -9.999999999999982236 ) ) ;
#8321=DIRECTION ( 'NONE',  ( 0.000000000000000000, -1.000000000000000000, 0.000000000000000000 ) ) ;
#8331=DIRECTION ( 'NONE',  ( 0.000000000000000000, 0.000000000000000000, -1.000000000000000000 ) ) ;
#8337=AXIS2_PLACEMENT_3D ( 'NONE', #13569, #20782, #4811 ) ;
#8341=EDGE_CURVE ( 'NONE', #21383, #3254, #5502, .T. ) ;
#8342=EDGE_CURVE ( 'NONE', #10602, #2469, #1842, .T. ) ;
#8344=DIRECTION ( 'NONE',  ( -1.458023040593674845E-16, 0.000000000000000000, -1.000000000000000000 ) ) ;
#8347=DIRECTION ( 'NONE',  ( 1.387778780781444256E-14, 0.000000000000000000, 1.000000000000000000 ) ) ;
#8349=DIRECTION ( 'NONE',  ( -6.938893903907215756E-15, 0.000000000000000000, 1.000000000000000000 ) ) ;
#8350=CARTESIAN_POINT ( 'NONE',  ( 163.9999999999998863, 18.00000000000000355, 8.000000000002229328 ) ) ;
#8364=DIRECTION ( 'NONE',  ( -0.4397038457472313144, 0.000000000000000000, -0.8981428216242086648 ) ) ;
#8372=ORIENTED_EDGE ( 'NONE', *, *, #2650, .T. ) ;
#8376=DIRECTION ( 'NONE',  ( -0.000000000000000000, -1.000000000000000000, 0.000000000000000000 ) ) ;
#8384=DIRECTION ( 'NONE',  ( -1.000000000000000000, 0.000000000000000000, 0.000000000000000000 ) ) ;
#8408=DIRECTION ( 'NONE',  ( 0.000000000000000000, 0.000000000000000000, 1.000000000000000000 ) ) ;
#8411=CARTESIAN_POINT ( 'NONE',  ( -158.3970384574724051, 1.999999999999998224, 62.74304228515463677 ) ) ;
#8419=AXIS2_PLACEMENT_3D ( 'NONE', #17110, #1375, #8349 ) ;
#8422=PLANE ( 'NONE',  #673 ) ;
#8432=CIRCLE ( 'NONE', #17626, 8.000000000000014211 ) ;
#8434=PRODUCT_DEFINITION_FORMATION_WITH_SPECIFIED_SOURCE ( 'ANY', '', #18346, .NOT_KNOWN. ) ;
#8436=AXIS2_PLACEMENT_3D ( 'NONE', #5807, #12841, #7435 ) ;
#8443=DIRECTION ( 'NONE',  ( -0.000000000000000000, -1.000000000000000000, -0.000000000000000000 ) ) ;
#8464=EDGE_LOOP ( 'NONE', ( #620, #3032, #4088, #19026 ) ) ;
#8468=CARTESIAN_POINT ( 'NONE',  ( -146.5000000000000000, 1.999999999999998224, 10.00000000000002487 ) ) ;
#8469=ORIENTED_EDGE ( 'NONE', *, *, #9794, .F. ) ;
#8471=CARTESIAN_POINT ( 'NONE',  ( 158.3970384574715808, 1.999999999999998224, 62.74304228515676130 ) ) ;
#8493=VECTOR ( 'NONE', #8443, 1000.000000000000000 ) ;
#8509=CARTESIAN_POINT ( 'NONE',  ( 158.3970384574715524, 20.00000000000000000, -62.74304228515679682 ) ) ;
#8510=DIRECTION ( 'NONE',  ( 0.000000000000000000, 1.000000000000000000, 0.000000000000000000 ) ) ;
#8518=ORIENTED_EDGE ( 'NONE', *, *, #9794, .T. ) ;
#8521=CARTESIAN_POINT ( 'NONE',  ( -55.40268456415260800, 1.999999999999998224, 113.1659955246496025 ) ) ;
#8530=EDGE_LOOP ( 'NONE', ( #11472, #11034, #3246, #4628 ) ) ;
#8538=DIRECTION ( 'NONE',  ( -0.000000000000000000, -1.000000000000000000, -0.000000000000000000 ) ) ;
#8540=DIRECTION ( 'NONE',  ( -0.000000000000000000, -1.000000000000000000, 0.000000000000000000 ) ) ;
#8541=CARTESIAN_POINT ( 'NONE',  ( 162.0000000000000000, 2.000000000000000000, 2.222801351277976832E-12 ) ) ;
#8551=ADVANCED_FACE ( 'NONE', ( #16198, #12503 ), #14581, .T. ) ;
#8554=VERTEX_POINT ( 'NONE', #5701 ) ;
#8562=CARTESIAN_POINT ( 'NONE',  ( 0.000000000000000000, 45.00000000000000000, 0.000000000000000000 ) ) ;
#8582=CARTESIAN_POINT ( 'NONE',  ( 163.1715728752537018, 20.00000000000000000, 8.828427124748406740 ) ) ;
#8591=EDGE_LOOP ( 'NONE', ( #12621, #14269, #16261, #19878 ) ) ;
#8602=VERTEX_POINT ( 'NONE', #9956 ) ;
#8607=CARTESIAN_POINT ( 'NONE',  ( 0.000000000000000000, 0.000000000000000000, 0.000000000000000000 ) ) ;
#8616=CIRCLE ( 'NONE', #16729, 124.0000000000000000 ) ;
#8625=ORIENTED_EDGE ( 'NONE', *, *, #11910, .T. ) ;
#8626=FACE_BOUND ( 'NONE', #8250, .T. ) ;
#8642=DIRECTION ( 'NONE',  ( -0.000000000000000000, -1.000000000000000000, -0.000000000000000000 ) ) ;
#8646=PLANE ( 'NONE',  #17262 ) ;
#8649=LINE ( 'NONE', #10854, #7473 ) ;
#8663=ADVANCED_FACE ( 'NONE', ( #21870 ), #21762, .F. ) ;
#8682=CARTESIAN_POINT ( 'NONE',  ( -90.00000000000000000, 29.00000000000000355, 8.394090934816448357E-16 ) ) ;
#8687=AXIS2_PLACEMENT_3D ( 'NONE', #13028, #21483, #4141 ) ;
#8697=ORIENTED_EDGE ( 'NONE', *, *, #19180, .T. ) ;
#8707=ORIENTED_EDGE ( 'NONE', *, *, #585, .T. ) ;
#8708=CARTESIAN_POINT ( 'NONE',  ( 0.000000000000000000, 23.00000000000000000, 0.000000000000000000 ) ) ;
#8709=DIRECTION ( 'NONE',  ( -0.000000000000000000, -1.000000000000000000, -0.000000000000000000 ) ) ;
#8727=CYLINDRICAL_SURFACE ( 'NONE', #4155, 2.000000000000000000 ) ;
#8730=CARTESIAN_POINT ( 'NONE',  ( 0.000000000000000000, 0.000000000000000000, -96.00000000000000000 ) ) ;
#8737=CARTESIAN_POINT ( 'NONE',  ( 0.000000000000000000, 20.00000000000000000, 0.000000000000000000 ) ) ;
#8747=EDGE_LOOP ( 'NONE', ( #6439, #19681, #4573, #9927 ) ) ;
#8748=DIRECTION ( 'NONE',  ( 1.372099599554306628E-14, 0.000000000000000000, -1.000000000000000000 ) ) ;
#8749=DIRECTION ( 'NONE',  ( 0.000000000000000000, -1.000000000000000000, 0.000000000000000000 ) ) ;
#8777=TOROIDAL_SURFACE ( 'NONE', #16164, 8.000000000000014211, 2.000000000000000000 ) ;
#8783=EDGE_LOOP ( 'NONE', ( #13163, #8697, #10453, #10142 ) ) ;
#8797=EDGE_CURVE ( 'NONE', #3937, #2916, #15819, .T. ) ;
#8862=CARTESIAN_POINT ( 'NONE',  ( 164.0000000000000000, 1.999999999999998224, -2.290411758281096087E-12 ) ) ;
#8865=CARTESIAN_POINT ( 'NONE',  ( -90.00000000000000000, 0.000000000000000000, -10.99999999999999289 ) ) ;
#8879=CARTESIAN_POINT ( 'NONE',  ( 0.000000000000000000, 37.00000000000000711, -96.00000000000000000 ) ) ;
#8882=DIRECTION ( 'NONE',  ( 0.000000000000000000, 0.000000000000000000, -1.000000000000000000 ) ) ;
#8890=ORIENTED_EDGE ( 'NONE', *, *, #9966, .T. ) ;
#8891=LINE ( 'NONE', #21405, #2595 ) ;
#8892=AXIS2_PLACEMENT_3D ( 'NONE', #12637, #9035, #15981 ) ;
#8899=ORIENTED_EDGE ( 'NONE', *, *, #10599, .T. ) ;
#8917=VECTOR ( 'NONE', #5665, 1000.000000000000000 ) ;
#8926=AXIS2_PLACEMENT_3D ( 'NONE', #19341, #5663, #10614 ) ;
#8928=CIRCLE ( 'NONE', #8208, 96.00000000000000000 ) ;
#8935=CIRCLE ( 'NONE', #5249, 10.00000000000000888 ) ;
#8942=ORIENTED_EDGE ( 'NONE', *, *, #3252, .F. ) ;
#8951=ORIENTED_EDGE ( 'NONE', *, *, #6650, .F. ) ;
#8974=LINE ( 'NONE', #8730, #14097 ) ;
#9024=CARTESIAN_POINT ( 'NONE',  ( -163.1715728752537871, 20.00000000000000000, -8.828427124746170307 ) ) ;
#9035=DIRECTION ( 'NONE',  ( 0.000000000000000000, 0.000000000000000000, 1.000000000000000000 ) ) ;
#9038=VERTEX_POINT ( 'NONE', #525 ) ;
#9056=VERTEX_POINT ( 'NONE', #6137 ) ;
#9058=CARTESIAN_POINT ( 'NONE',  ( -54.52327687265817246, 18.00000000000000355, -111.3697098814011781 ) ) ;
#9064=VERTEX_POINT ( 'NONE', #1090 ) ;
#9091=EDGE_LOOP ( 'NONE', ( #4356, #15782, #7793, #6125 ) ) ;
#9117=DIRECTION ( 'NONE',  ( 0.000000000000000000, -0.000000000000000000, 1.000000000000000000 ) ) ;
#9118=ADVANCED_FACE ( 'NONE', ( #14786 ), #12941, .T. ) ;
#9167=DIRECTION ( 'NONE',  ( 0.8981428216242073326, 1.525529167390024815E-15, 0.4397038457472340900 ) ) ;
#9169=AXIS2_PLACEMENT_3D ( 'NONE', #12808, #9710, #16620 ) ;
#9181=CIRCLE ( 'NONE', #17276, 10.00000000000000355 ) ;
#9202=CYLINDRICAL_SURFACE ( 'NONE', #5964, 2.000000000000000000 ) ;
#9203=CARTESIAN_POINT ( 'NONE',  ( 1.457329690985350156E-14, 25.00000000000000000, -118.0000000000000000 ) ) ;
#9204=DIRECTION ( 'NONE',  ( 0.000000000000000000, 1.000000000000000000, -0.000000000000000000 ) ) ;
#9206=ORIENTED_EDGE ( 'NONE', *, *, #12655, .T. ) ;
#9211=VERTEX_POINT ( 'NONE', #4630 ) ;
#9219=ADVANCED_FACE ( 'NONE', ( #16950 ), #1214, .T. ) ;
#9224=VECTOR ( 'NONE', #22621, 1000.000000000000000 ) ;
#9255=ORIENTED_EDGE ( 'NONE', *, *, #21675, .F. ) ;
#9263=CARTESIAN_POINT ( 'NONE',  ( -164.0000000000000284, 19.17157287525381193, -7.999999999999978684 ) ) ;
#9271=ORIENTED_EDGE ( 'NONE', *, *, #18630, .T. ) ;
#9276=AXIS2_PLACEMENT_3D ( 'NONE', #8708, #21019, #3666 ) ;
#9282=EDGE_CURVE ( 'NONE', #6252, #21740, #4268, .T. ) ;
#9287=EDGE_LOOP ( 'NONE', ( #6814, #19497, #11577, #8942 ) ) ;
#9292=CARTESIAN_POINT ( 'NONE',  ( 153.9999999999992610, 1.999999999999998224, 53.76161406891468175 ) ) ;
#9299=CARTESIAN_POINT ( 'NONE',  ( -164.0000000000000000, 1.999999999999998224, 8.000000000000019540 ) ) ;
#9307=EDGE_LOOP ( 'NONE', ( #10889, #14397, #20747, #4894 ) ) ;
#9308=DIRECTION ( 'NONE',  ( 2.449293598294706414E-16, 0.000000000000000000, 1.000000000000000000 ) ) ;
#9322=AXIS2_PLACEMENT_3D ( 'NONE', #21702, #5867, #14865 ) ;
#9323=DIRECTION ( 'NONE',  ( 0.000000000000000000, 0.000000000000000000, 1.000000000000000000 ) ) ;
#9325=CARTESIAN_POINT ( 'NONE',  ( 0.000000000000000000, 25.00000000000000000, 0.000000000000000000 ) ) ;
#9333=CARTESIAN_POINT ( 'NONE',  ( 0.000000000000000000, 18.00000000000000355, 0.000000000000000000 ) ) ;
#9344=AXIS2_PLACEMENT_3D ( 'NONE', #8468, #2859, #18702 ) ;
#9372=DIRECTION ( 'NONE',  ( 1.000000000000000000, 0.000000000000000000, 0.000000000000000000 ) ) ;
#9381=ORIENTED_EDGE ( 'NONE', *, *, #1523, .T. ) ;
#9387=ORIENTED_EDGE ( 'NONE', *, *, #22270, .F. ) ;
#9389=ADVANCED_FACE ( 'NONE', ( #17907 ), #16583, .T. ) ;
#9391=DIRECTION ( 'NONE',  ( -1.387778780781445202E-14, 0.000000000000000000, 1.000000000000000000 ) ) ;
#9394=ORIENTED_EDGE ( 'NONE', *, *, #3596, .T. ) ;
#9399=ORIENTED_EDGE ( 'NONE', *, *, #475, .F. ) ;
#9403=VERTEX_POINT ( 'NONE', #15455 ) ;
#9405=CARTESIAN_POINT ( 'NONE',  ( -54.52327687265817957, 2.000000000000000000, -111.3697098814011923 ) ) ;
#9406=EDGE_CURVE ( 'NONE', #3408, #7438, #19475, .T. ) ;
#9416=VERTEX_POINT ( 'NONE', #19814 ) ;
#9417=CARTESIAN_POINT ( 'NONE',  ( -162.0000000000000000, 20.00000000000000000, -9.999999999999978684 ) ) ;
#9427=DIRECTION ( 'NONE',  ( 0.000000000000000000, 1.000000000000000000, -0.000000000000000000 ) ) ;
#9428=DIRECTION ( 'NONE',  ( -2.449293598294706414E-16, 0.000000000000000000, -1.000000000000000000 ) ) ;
#9434=ORIENTED_EDGE ( 'NONE', *, *, #17945, .T. ) ;
#9451=DIRECTION ( 'NONE',  ( 0.000000000000000000, 0.000000000000000000, 1.000000000000000000 ) ) ;
#9467=ORIENTED_EDGE ( 'NONE', *, *, #18951, .F. ) ;
#9487=CARTESIAN_POINT ( 'NONE',  ( 0.000000000000000000, 0.000000000000000000, 0.000000000000000000 ) ) ;
#9506=AXIS2_PLACEMENT_3D ( 'NONE', #2652, #7923, #14956 ) ;
#9544=VECTOR ( 'NONE', #8044, 1000.000000000000114 ) ;
#9545=CARTESIAN_POINT ( 'NONE',  ( 153.9999999999992610, 1.999999999999998224, -53.76161406891471017 ) ) ;
#9555=ORIENTED_EDGE ( 'NONE', *, *, #11609, .T. ) ;
#9558=AXIS2_PLACEMENT_3D ( 'NONE', #17452, #13879, #1590 ) ;
#9582=DIRECTION ( 'NONE',  ( 0.000000000000000000, 1.000000000000000000, -0.000000000000000000 ) ) ;
#9587=DIRECTION ( 'NONE',  ( 0.8981428216242033358, 0.000000000000000000, -0.4397038457472424167 ) ) ;
#9593=CARTESIAN_POINT ( 'NONE',  ( 0.000000000000000000, 0.000000000000000000, 0.000000000000000000 ) ) ;
#9599=VERTEX_POINT ( 'NONE', #8865 ) ;
#9602=CYLINDRICAL_SURFACE ( 'NONE', #6172, 2.000000000000001332 ) ;
#9605=CARTESIAN_POINT ( 'NONE',  ( 163.1715728752537018, -1.082576183735519500E-15, -8.828427124748447596 ) ) ;
#9620=AXIS2_PLACEMENT_3D ( 'NONE', #11623, #22370, #1398 ) ;
#9641=CARTESIAN_POINT ( 'NONE',  ( 157.5176307659770885, 0.000000000000000000, -60.94675664190840081 ) ) ;
#9642=EDGE_CURVE ( 'NONE', #17220, #99, #2552, .T. ) ;
#9645=FACE_OUTER_BOUND ( 'NONE', #19143, .T. ) ;
#9647=ORIENTED_EDGE ( 'NONE', *, *, #11041, .F. ) ;
#9657=EDGE_CURVE ( 'NONE', #7993, #10504, #21447, .T. ) ;
#9662=DIRECTION ( 'NONE',  ( 0.4397038457472313144, 0.000000000000000000, -0.8981428216242086648 ) ) ;
#9674=DIRECTION ( 'NONE',  ( 1.000000000000000000, -0.000000000000000000, 1.362186893977296347E-14 ) ) ;
#9679=SURFACE_SIDE_STYLE ('',( #22164 ) ) ;
#9695=CYLINDRICAL_SURFACE ( 'NONE', #11462, 10.00000000000001599 ) ;
#9702=ORIENTED_EDGE ( 'NONE', *, *, #10996, .F. ) ;
#9710=DIRECTION ( 'NONE',  ( -0.4397038457472309814, 0.000000000000000000, -0.8981428216242088869 ) ) ;
#9724=AXIS2_PLACEMENT_3D ( 'NONE', #17458, #13777, #3298 ) ;
#9730=( BOUNDED_CURVE ( )  B_SPLINE_CURVE ( 3, ( #19147, #8582, #6856, #8350 ),
 .UNSPECIFIED., .F., .T. ) 
 B_SPLINE_CURVE_WITH_KNOTS ( ( 4, 4 ),
 ( 1.570796326794896558, 3.141592653589793116 ),
 .UNSPECIFIED. ) 
 CURVE ( )  GEOMETRIC_REPRESENTATION_ITEM ( )  RATIONAL_B_SPLINE_CURVE ( ( 1.000000000000000000, 0.8047378541243649375, 0.8047378541243649375, 1.000000000000000000 ) ) 
 REPRESENTATION_ITEM ( '' )  );
#9737=DIRECTION ( 'NONE',  ( -0.4397038457472424167, 0.000000000000000000, 0.8981428216242032248 ) ) ;
#9740=VERTEX_POINT ( 'NONE', #12684 ) ;
#9750=CARTESIAN_POINT ( 'NONE',  ( -164.0000000000000000, 20.00000000000000000, -7.999999999999979572 ) ) ;
#9753=ORIENTED_EDGE ( 'NONE', *, *, #15175, .F. ) ;
#9756=CARTESIAN_POINT ( 'NONE',  ( -146.5000000000000000, 18.00000000000000355, 2.081668171172168513E-14 ) ) ;
#9760=VERTEX_POINT ( 'NONE', #9203 ) ;
#9780=ORIENTED_EDGE ( 'NONE', *, *, #17432, .F. ) ;
#9782=CARTESIAN_POINT ( 'NONE',  ( 0.000000000000000000, 0.000000000000000000, 0.000000000000000000 ) ) ;
#9794=EDGE_CURVE ( 'NONE', #3243, #19859, #1296, .T. ) ;
#9835=EDGE_CURVE ( 'NONE', #17029, #7846, #11941, .T. ) ;
#9842=ORIENTED_EDGE ( 'NONE', *, *, #1776, .F. ) ;
#9845=MANIFOLD_SOLID_BREP ( 'Stock-MAS-425-1', #5595 ) ;
#9846=CIRCLE ( 'NONE', #1782, 8.000000000000014211 ) ;
#9851=AXIS2_PLACEMENT_3D ( 'NONE', #9884, #8166, #15199 ) ;
#9863=ORIENTED_EDGE ( 'NONE', *, *, #14997, .T. ) ;
#9878=DIRECTION ( 'NONE',  ( 0.000000000000000000, 0.000000000000000000, 1.000000000000000000 ) ) ;
#9884=CARTESIAN_POINT ( 'NONE',  ( -90.00000000000000000, 29.00000000000000355, 8.394090934816448357E-16 ) ) ;
#9891=EDGE_CURVE ( 'NONE', #20163, #17220, #14871, .T. ) ;
#9910=CARTESIAN_POINT ( 'NONE',  ( 0.000000000000000000, 20.00000000000000000, 0.000000000000000000 ) ) ;
#9912=CARTESIAN_POINT ( 'NONE',  ( 0.000000000000000000, 18.00000000000000355, 0.000000000000000000 ) ) ;
#9920=EDGE_CURVE ( 'NONE', #10082, #19973, #7160, .T. ) ;
#9925=DIRECTION ( 'NONE',  ( 1.000000000000000000, 0.000000000000000000, -1.396592535537260757E-14 ) ) ;
#9926=CARTESIAN_POINT ( 'NONE',  ( 153.9999999999992610, 20.00000000000000000, 53.76161406891468175 ) ) ;
#9927=ORIENTED_EDGE ( 'NONE', *, *, #10461, .F. ) ;
#9928=CARTESIAN_POINT ( 'NONE',  ( -146.5000000000000000, 0.000000000000000000, -9.999999999999982236 ) ) ;
#9931=DIRECTION ( 'NONE',  ( -0.4397038457472429718, 0.000000000000000000, 0.8981428216242028917 ) ) ;
#9940=AXIS2_PLACEMENT_3D ( 'NONE', #21077, #9117, #1786 ) ;
#9941=DIRECTION ( 'NONE',  ( -0.4397038457472479678, 0.000000000000000000, -0.8981428216242003382 ) ) ;
#9944=CARTESIAN_POINT ( 'NONE',  ( 1.458023040593674057E-15, 18.00000000000000355, 9.999999999999994671 ) ) ;
#9948=EDGE_CURVE ( 'NONE', #3348, #15608, #12196, .T. ) ;
#9949=DIRECTION ( 'NONE',  ( 0.000000000000000000, 0.000000000000000000, -1.000000000000000000 ) ) ;
#9954=VERTEX_POINT ( 'NONE', #10127 ) ;
#9956=CARTESIAN_POINT ( 'NONE',  ( -158.3970384574724335, 1.999999999999998224, -62.74304228515459414 ) ) ;
#9958=ORIENTED_EDGE ( 'NONE', *, *, #17387, .F. ) ;
#9962=AXIS2_PLACEMENT_3D ( 'NONE', #22489, #8051, #4492 ) ;
#9966=EDGE_CURVE ( 'NONE', #19051, #16346, #10353, .T. ) ;
#9977=CONICAL_SURFACE ( 'NONE', #820, 117.0000000000000000, 0.3316125578789227979 ) ;
#9987=CARTESIAN_POINT ( 'NONE',  ( -9.912705577010314703E-16, 0.000000000000000000, -9.999999999999994671 ) ) ;
#9991=EDGE_CURVE ( 'NONE', #18579, #7906, #15993, .T. ) ;
#9996=ORIENTED_EDGE ( 'NONE', *, *, #8797, .T. ) ;
#10006=DIRECTION ( 'NONE',  ( 1.387778780781444571E-14, -0.000000000000000000, 1.000000000000000000 ) ) ;
#10007=DIRECTION ( 'NONE',  ( 0.8981428216242060003, 1.398976466700252608E-14, 0.4397038457472368655 ) ) ;
#10009=CARTESIAN_POINT ( 'NONE',  ( -79.00000000000000000, 29.00000000000000355, 7.368146487227772848E-16 ) ) ;
#10010=CIRCLE ( 'NONE', #10746, 124.0000000000000000 ) ;
#10012=EDGE_LOOP ( 'NONE', ( #5274, #3903 ) ) ;
#10014=FILL_AREA_STYLE_COLOUR ( '', #17455 ) ;
#10032=CYLINDRICAL_SURFACE ( 'NONE', #19193, 2.000000000000000000 ) ;
#10037=VECTOR ( 'NONE', #1344, 1000.000000000000000 ) ;
#10043=VECTOR ( 'NONE', #1978, 1000.000000000000000 ) ;
#10051=EDGE_CURVE ( 'NONE', #7993, #22518, #8616, .T. ) ;
#10053=VECTOR ( 'NONE', #9674, 1000.000000000000000 ) ;
#10064=DIRECTION ( 'NONE',  ( 0.000000000000000000, 0.000000000000000000, 1.000000000000000000 ) ) ;
#10067=DIRECTION ( 'NONE',  ( 1.458023040593674845E-16, 0.000000000000000000, 1.000000000000000000 ) ) ;
#10082=VERTEX_POINT ( 'NONE', #2297 ) ;
#10094=CYLINDRICAL_SURFACE ( 'NONE', #12557, 2.000000000000000000 ) ;
#10107=EDGE_CURVE ( 'NONE', #9038, #18453, #924, .T. ) ;
#10109=DIRECTION ( 'NONE',  ( 0.000000000000000000, -1.000000000000000000, 0.000000000000000000 ) ) ;
#10110=VERTEX_POINT ( 'NONE', #7913 ) ;
#10115=CARTESIAN_POINT ( 'NONE',  ( -55.40268456415261511, 18.00000000000000355, 113.1659955246496025 ) ) ;
#10121=CARTESIAN_POINT ( 'NONE',  ( 157.5176307659771453, 20.00000000000000000, 60.94675664190832975 ) ) ;
#10122=DIRECTION ( 'NONE',  ( -0.8981428216242087759, 0.000000000000000000, 0.4397038457472309259 ) ) ;
#10127=CARTESIAN_POINT ( 'NONE',  ( -90.00000000000000000, 29.00000000000000355, 10.99999999999999289 ) ) ;
#10129=ORIENTED_EDGE ( 'NONE', *, *, #19159, .T. ) ;
#10142=ORIENTED_EDGE ( 'NONE', *, *, #11041, .T. ) ;
#10158=ORIENTED_EDGE ( 'NONE', *, *, #4774, .F. ) ;
#10161=DIRECTION ( 'NONE',  ( -2.449293598294706414E-16, 0.000000000000000000, -1.000000000000000000 ) ) ;
#10166=DIRECTION ( 'NONE',  ( 1.224646799147349509E-16, 0.000000000000000000, -1.000000000000000000 ) ) ;
#10170=ORIENTED_EDGE ( 'NONE', *, *, #2689, .F. ) ;
#10172=ORIENTED_EDGE ( 'NONE', *, *, #3141, .T. ) ;
#10199=VERTEX_POINT ( 'NONE', #13105 ) ;
#10233=VERTEX_POINT ( 'NONE', #3224 ) ;
#10236=CARTESIAN_POINT ( 'NONE',  ( 0.000000000000000000, 18.00000000000000355, 0.000000000000000000 ) ) ;
#10244=EDGE_LOOP ( 'NONE', ( #17095, #139, #13900, #7421 ) ) ;
#10245=CARTESIAN_POINT ( 'NONE',  ( 3.086109933851330151E-14, 18.00000000000000355, 126.0000000000000000 ) ) ;
#10261=ORIENTED_EDGE ( 'NONE', *, *, #14466, .F. ) ;
#10280=EDGE_LOOP ( 'NONE', ( #2030, #6706, #4524, #13031 ) ) ;
#10287=CIRCLE ( 'NONE', #2581, 2.000000000000000000 ) ;
#10293=CARTESIAN_POINT ( 'NONE',  ( -54.52327687265812983, 0.000000000000000000, 111.3697098814011923 ) ) ;
#10300=DIRECTION ( 'NONE',  ( 0.000000000000000000, -0.000000000000000000, 1.000000000000000000 ) ) ;
#10308=ORIENTED_EDGE ( 'NONE', *, *, #22655, .F. ) ;
#10333=EDGE_CURVE ( 'NONE', #7846, #15942, #19635, .T. ) ;
#10349=LINE ( 'NONE', #18613, #5776 ) ;
#10353=LINE ( 'NONE', #19179, #17084 ) ;
#10355=CIRCLE ( 'NONE', #9620, 96.00000000000000000 ) ;
#10357=AXIS2_PLACEMENT_3D ( 'NONE', #2620, #14592, #16324 ) ;
#10360=ORIENTED_EDGE ( 'NONE', *, *, #15886, .T. ) ;
#10364=CARTESIAN_POINT ( 'NONE',  ( -7.930164461608248607E-16, 1.999999999999998224, -7.999999999999994671 ) ) ;
#10366=EDGE_CURVE ( 'NONE', #10110, #15997, #21820, .T. ) ;
#10381=CARTESIAN_POINT ( 'NONE',  ( 0.000000000000000000, 20.00000000000000000, 0.000000000000000000 ) ) ;
#10398=LINE ( 'NONE', #4641, #3788 ) ;
#10412=AXIS2_PLACEMENT_3D ( 'NONE', #16725, #867, #16491 ) ;
#10419=DIRECTION ( 'NONE',  ( -0.000000000000000000, -1.000000000000000000, -0.000000000000000000 ) ) ;
#10424=VECTOR ( 'NONE', #10489, 1000.000000000000000 ) ;
#10440=TOROIDAL_SURFACE ( 'NONE', #545, 10.00000000000000355, 2.000000000000000000 ) ;
#10442=CARTESIAN_POINT ( 'NONE',  ( 0.000000000000000000, 25.00000000000000000, 117.0000000000000000 ) ) ;
#10443=CARTESIAN_POINT ( 'NONE',  ( 0.000000000000000000, 25.00000000000000000, 117.0000000000000000 ) ) ;
#10449=CARTESIAN_POINT ( 'NONE',  ( -54.52327687265812273, 20.00000000000000000, 111.3697098814011923 ) ) ;
#10451=DIRECTION ( 'NONE',  ( 0.000000000000000000, 1.000000000000000000, -0.000000000000000000 ) ) ;
#10453=ORIENTED_EDGE ( 'NONE', *, *, #1551, .F. ) ;
#10461=EDGE_CURVE ( 'NONE', #19256, #11124, #10856, .T. ) ;
#10464=DIRECTION ( 'NONE',  ( -1.000000000000000000, 0.000000000000000000, 1.458023040593674599E-16 ) ) ;
#10469=ORIENTED_EDGE ( 'NONE', *, *, #17387, .T. ) ;
#10479=CARTESIAN_POINT ( 'NONE',  ( 54.52327687265663769, 18.00000000000000355, 111.3697098814019171 ) ) ;
#10488=VERTEX_POINT ( 'NONE', #20540 ) ;
#10489=DIRECTION ( 'NONE',  ( -0.000000000000000000, -1.000000000000000000, -0.000000000000000000 ) ) ;
#10504=VERTEX_POINT ( 'NONE', #10115 ) ;
#10510=CARTESIAN_POINT ( 'NONE',  ( 164.0000000000000000, 20.00000000000000000, -2.290411758281096087E-12 ) ) ;
#10513=CARTESIAN_POINT ( 'NONE',  ( 0.000000000000000000, 1.999999999999998224, 0.000000000000000000 ) ) ;
#10549=DIRECTION ( 'NONE',  ( -2.449293598294706414E-16, -0.000000000000000000, -1.000000000000000000 ) ) ;
#10550=AXIS2_PLACEMENT_3D ( 'NONE', #6100, #4024, #9323 ) ;
#10551=LINE ( 'NONE', #15860, #14792 ) ;
#10556=EDGE_CURVE ( 'NONE', #99, #5930, #19280, .T. ) ;
#10560=EDGE_LOOP ( 'NONE', ( #19740, #15680, #7382, #16065 ) ) ;
#10562=CARTESIAN_POINT ( 'NONE',  ( 158.3970384574715524, 1.999999999999998224, -62.74304228515679682 ) ) ;
#10579=ORIENTED_EDGE ( 'NONE', *, *, #6954, .F. ) ;
#10585=ORIENTED_EDGE ( 'NONE', *, *, #9406, .T. ) ;
#10586=DIRECTION ( 'NONE',  ( -1.000000000000000000, 0.000000000000000000, 0.000000000000000000 ) ) ;
#10599=EDGE_CURVE ( 'NONE', #14514, #17969, #4239, .T. ) ;
#10600=DIRECTION ( 'NONE',  ( 0.000000000000000000, 1.000000000000000000, -0.000000000000000000 ) ) ;
#10602=VERTEX_POINT ( 'NONE', #17703 ) ;
#10614=DIRECTION ( 'NONE',  ( -0.8981428216242027807, 0.000000000000000000, 0.4397038457472431938 ) ) ;
#10646=CARTESIAN_POINT ( 'NONE',  ( 146.5000000000000000, 18.00000000000000355, -2.025191382850354537E-12 ) ) ;
#10647=CARTESIAN_POINT ( 'NONE',  ( -164.0000000000000000, 20.00000000000000000, 8.000000000000019540 ) ) ;
#10670=VECTOR ( 'NONE', #12445, 1000.000000000000000 ) ;
#10671=ORIENTED_EDGE ( 'NONE', *, *, #6348, .F. ) ;
#10673=DIRECTION ( 'NONE',  ( 0.000000000000000000, 0.000000000000000000, 1.000000000000000000 ) ) ;
#10676=EDGE_LOOP ( 'NONE', ( #8022, #3023, #19941, #18989 ) ) ;
#10678=ORIENTED_EDGE ( 'NONE', *, *, #1241, .T. ) ;
#10683=ORIENTED_EDGE ( 'NONE', *, *, #6427, .T. ) ;
#10684=DIRECTION ( 'NONE',  ( 0.000000000000000000, 1.000000000000000000, -0.000000000000000000 ) ) ;
#10688=EDGE_CURVE ( 'NONE', #1991, #3937, #12304, .T. ) ;
#10705=VERTEX_POINT ( 'NONE', #3546 ) ;
#10707=VERTEX_POINT ( 'NONE', #10562 ) ;
#10708=CARTESIAN_POINT ( 'NONE',  ( -162.0000000000000000, 20.00000000000000000, 10.00000000000001954 ) ) ;
#10732=CARTESIAN_POINT ( 'NONE',  ( 157.5176307659771169, 18.00000000000000355, 60.94675664190834397 ) ) ;
#10735=CARTESIAN_POINT ( 'NONE',  ( 0.000000000000000000, 45.00000000000000711, 0.000000000000000000 ) ) ;
#10736=EDGE_CURVE ( 'NONE', #22518, #2811, #972, .T. ) ;
#10746=AXIS2_PLACEMENT_3D ( 'NONE', #20171, #2506, #5946 ) ;
#10751=VERTEX_POINT ( 'NONE', #4198 ) ;
#10763=EDGE_LOOP ( 'NONE', ( #20452, #4775 ) ) ;
#10766=CARTESIAN_POINT ( 'NONE',  ( -54.52327687265813694, 20.00000000000000000, 111.3697098814011781 ) ) ;
#10808=CARTESIAN_POINT ( 'NONE',  ( -162.0000000000000000, 18.00000000000000355, 0.000000000000000000 ) ) ;
#10812=ORIENTED_EDGE ( 'NONE', *, *, #13167, .F. ) ;
#10831=ORIENTED_EDGE ( 'NONE', *, *, #19326, .T. ) ;
#10838=EDGE_LOOP ( 'NONE', ( #21622, #8118, #21031, #7239, #9399 ) ) ;
#10849=DIRECTION ( 'NONE',  ( 0.8981428216242066664, 0.000000000000000000, -0.4397038457472354778 ) ) ;
#10852=DIRECTION ( 'NONE',  ( 0.000000000000000000, 0.000000000000000000, 1.000000000000000000 ) ) ;
#10854=CARTESIAN_POINT ( 'NONE',  ( 55.40268456415108034, 18.00000000000000355, 113.1659955246503557 ) ) ;
#10856=CIRCLE ( 'NONE', #18211, 10.00000000000000355 ) ;
#10857=DIRECTION ( 'NONE',  ( 0.000000000000000000, 1.000000000000000000, -0.000000000000000000 ) ) ;
#10864=ORIENTED_EDGE ( 'NONE', *, *, #15975, .T. ) ;
#10873=ORIENTED_EDGE ( 'NONE', *, *, #10333, .F. ) ;
#10883=CARTESIAN_POINT ( 'NONE',  ( 161.9999999999992610, 18.00000000000000355, 53.76161406891478123 ) ) ;
#10889=ORIENTED_EDGE ( 'NONE', *, *, #172, .T. ) ;
#10892=ORIENTED_EDGE ( 'NONE', *, *, #12423, .T. ) ;
#10901=ORIENTED_EDGE ( 'NONE', *, *, #9991, .T. ) ;
#10903=CARTESIAN_POINT ( 'NONE',  ( 161.9999999999998579, 0.000000000000000000, -10.00000000000224176 ) ) ;
#10918=EDGE_CURVE ( 'NONE', #21383, #17288, #8227, .T. ) ;
#10929=CIRCLE ( 'NONE', #8337, 118.0000000000000000 ) ;
#10970=AXIS2_PLACEMENT_3D ( 'NONE', #13437, #20519, #4779 ) ;
#10983=LINE ( 'NONE', #7426, #19224 ) ;
#10996=EDGE_CURVE ( 'NONE', #6260, #15641, #4526, .T. ) ;
#11009=CARTESIAN_POINT ( 'NONE',  ( -90.00000000000000000, 0.000000000000000000, 8.394090934816448357E-16 ) ) ;
#11024=CYLINDRICAL_SURFACE ( 'NONE', #21962, 2.000000000000001332 ) ;
#11029=DIRECTION ( 'NONE',  ( 0.000000000000000000, 0.000000000000000000, 1.000000000000000000 ) ) ;
#11030=ADVANCED_FACE ( 'NONE', ( #12122 ), #5996, .T. ) ;
#11034=ORIENTED_EDGE ( 'NONE', *, *, #632, .F. ) ;
#11041=EDGE_CURVE ( 'NONE', #9056, #10110, #17476, .T. ) ;
#11049=DIRECTION ( 'NONE',  ( -0.000000000000000000, -1.000000000000000000, -0.000000000000000000 ) ) ;
#11055=EDGE_CURVE ( 'NONE', #8554, #14680, #6017, .T. ) ;
#11060=ORIENTED_EDGE ( 'NONE', *, *, #5387, .T. ) ;
#11065=AXIS2_PLACEMENT_3D ( 'NONE', #12807, #19780, #8076 ) ;
#11099=AXIS2_PLACEMENT_3D ( 'NONE', #16694, #6203, #9878 ) ;
#11100=DIRECTION ( 'NONE',  ( 0.4397038457472424167, 0.000000000000000000, -0.8981428216242032248 ) ) ;
#11102=CARTESIAN_POINT ( 'NONE',  ( -55.40268456415261511, 20.00000000000000000, 113.1659955246496025 ) ) ;
#11107=ORIENTED_EDGE ( 'NONE', *, *, #17945, .F. ) ;
#11115=ADVANCED_FACE ( 'NONE', ( #2696 ), #2224, .T. ) ;
#11124=VERTEX_POINT ( 'NONE', #2574 ) ;
#11125=ORIENTED_EDGE ( 'NONE', *, *, #4242, .F. ) ;
#11127=AXIS2_PLACEMENT_3D ( 'NONE', #6498, #12005, #9941 ) ;
#11141=DIRECTION ( 'NONE',  ( -1.000000000000000000, 0.000000000000000000, 0.000000000000000000 ) ) ;
#11149=EDGE_LOOP ( 'NONE', ( #6024, #4378, #10812, #2711 ) ) ;
#11157=ORIENTED_EDGE ( 'NONE', *, *, #170, .T. ) ;
#11159=DIRECTION ( 'NONE',  ( -1.000000000000000000, 0.000000000000000000, 0.000000000000000000 ) ) ;
#11164=ORIENTED_EDGE ( 'NONE', *, *, #11817, .F. ) ;
#11169=DIRECTION ( 'NONE',  ( 0.000000000000000000, 0.000000000000000000, 1.000000000000000000 ) ) ;
#11172=VERTEX_POINT ( 'NONE', #4052 ) ;
#11203=CARTESIAN_POINT ( 'NONE',  ( -54.52327687265816536, 2.000000000000000000, -111.3697098814011923 ) ) ;
#11206=PRODUCT_DEFINITION_SHAPE ( 'NONE', 'NONE',  #2137 ) ;
#11210=CARTESIAN_POINT ( 'NONE',  ( 0.000000000000000000, 1.999999999999998224, 0.000000000000000000 ) ) ;
#11232=CARTESIAN_POINT ( 'NONE',  ( -54.52327687265816536, 0.000000000000000000, -111.3697098814011923 ) ) ;
#11256=ORIENTED_EDGE ( 'NONE', *, *, #6195, .T. ) ;
#11260=DIRECTION ( 'NONE',  ( 0.8981428216242028917, -0.000000000000000000, -0.4397038457472432493 ) ) ;
#11267=CYLINDRICAL_SURFACE ( 'NONE', #21327, 2.000000000000000000 ) ;
#11271=DIRECTION ( 'NONE',  ( 0.000000000000000000, 0.000000000000000000, 1.000000000000000000 ) ) ;
#11274=CYLINDRICAL_SURFACE ( 'NONE', #8007, 96.00000000000000000 ) ;
#11280=AXIS2_PLACEMENT_3D ( 'NONE', #7253, #9427, #605 ) ;
#11306=AXIS2_PLACEMENT_3D ( 'NONE', #20346, #13367, #8384 ) ;
#11319=EDGE_CURVE ( 'NONE', #19859, #3243, #13002, .T. ) ;
#11328=CARTESIAN_POINT ( 'NONE',  ( 1.175660927181459158E-14, 45.00000000000000711, 96.00000000000000000 ) ) ;
#11331=DIRECTION ( 'NONE',  ( 0.000000000000000000, 1.000000000000000000, 0.000000000000000000 ) ) ;
#11332=EDGE_CURVE ( 'NONE', #10488, #8008, #19203, .T. ) ;
#11334=LINE ( 'NONE', #6399, #16267 ) ;
#11356=FACE_OUTER_BOUND ( 'NONE', #13576, .T. ) ;
#11364=CIRCLE ( 'NONE', #13572, 10.99999999999999289 ) ;
#11367=ORIENTED_EDGE ( 'NONE', *, *, #1784, .T. ) ;
#11374=DIRECTION ( 'NONE',  ( 0.000000000000000000, 0.000000000000000000, -1.000000000000000000 ) ) ;
#11378=CARTESIAN_POINT ( 'NONE',  ( 1.469576158976823671E-14, 20.00000000000000000, 120.0000000000000000 ) ) ;
#11392=( NAMED_UNIT ( * ) SI_UNIT ( $, .STERADIAN. ) SOLID_ANGLE_UNIT ( ) );
#11399=CIRCLE ( 'NONE', #11, 2.000000000000001332 ) ;
#11417=CARTESIAN_POINT ( 'NONE',  ( -146.5000000000000000, 18.00000000000000355, 8.000000000000015987 ) ) ;
#11423=VECTOR ( 'NONE', #1617, 1000.000000000000114 ) ;
#11427=DIRECTION ( 'NONE',  ( 0.000000000000000000, 0.000000000000000000, -1.000000000000000000 ) ) ;
#11439=AXIS2_PLACEMENT_3D ( 'NONE', #10479, #17491, #16012 ) ;
#11446=LINE ( 'NONE', #11566, #11541 ) ;
#11458=EDGE_CURVE ( 'NONE', #16242, #2134, #8974, .T. ) ;
#11462=AXIS2_PLACEMENT_3D ( 'NONE', #966, #6233, #13259 ) ;
#11472=ORIENTED_EDGE ( 'NONE', *, *, #13167, .T. ) ;
#11477=ORIENTED_EDGE ( 'NONE', *, *, #3743, .T. ) ;
#11487=CIRCLE ( 'NONE', #20993, 10.00000000000000355 ) ;
#11491=ORIENTED_EDGE ( 'NONE', *, *, #17570, .T. ) ;
#11493=FACE_OUTER_BOUND ( 'NONE', #3320, .T. ) ;
#11501=DIRECTION ( 'NONE',  ( 1.372099599554306628E-14, -0.000000000000000000, -1.000000000000000000 ) ) ;
#11529=EDGE_CURVE ( 'NONE', #9038, #14045, #15209, .T. ) ;
#11532=ORIENTED_EDGE ( 'NONE', *, *, #3743, .F. ) ;
#11541=VECTOR ( 'NONE', #15023, 1000.000000000000000 ) ;
#11544=DIRECTION ( 'NONE',  ( -1.000000000000000000, 0.000000000000000000, 1.387778780781445676E-14 ) ) ;
#11563=CARTESIAN_POINT ( 'NONE',  ( 153.9999999999992610, 18.00000000000000355, 53.76161406891468175 ) ) ;
#11566=CARTESIAN_POINT ( 'NONE',  ( 163.9999999999998863, 18.00000000000000355, -8.000000000002268408 ) ) ;
#11577=ORIENTED_EDGE ( 'NONE', *, *, #17648, .F. ) ;
#11587=ORIENTED_EDGE ( 'NONE', *, *, #5139, .F. ) ;
#11599=CARTESIAN_POINT ( 'NONE',  ( 146.4999999999998863, 18.00000000000000355, 8.000000000001989520 ) ) ;
#11601=EDGE_LOOP ( 'NONE', ( #17356, #15255, #2334, #8190 ) ) ;
#11607=EDGE_CURVE ( 'NONE', #16346, #16446, #13379, .T. ) ;
#11609=EDGE_CURVE ( 'NONE', #10751, #9211, #8935, .T. ) ;
#11615=LINE ( 'NONE', #3196, #5368 ) ;
#11623=CARTESIAN_POINT ( 'NONE',  ( 0.000000000000000000, 37.00000000000000711, 0.000000000000000000 ) ) ;
#11625=DIRECTION ( 'NONE',  ( 1.372099599554306628E-14, -0.000000000000000000, -1.000000000000000000 ) ) ;
#11629=EDGE_CURVE ( 'NONE', #3254, #6576, #18722, .T. ) ;
#11645=AXIS2_PLACEMENT_3D ( 'NONE', #16901, #1169, #15072 ) ;
#11652=( NAMED_UNIT ( * ) PLANE_ANGLE_UNIT ( ) SI_UNIT ( $, .RADIAN. ) );
#11661=PLANE ( 'NONE',  #18156 ) ;
#11683=EDGE_CURVE ( 'NONE', #2811, #10705, #8169, .T. ) ;
#11693=CARTESIAN_POINT ( 'NONE',  ( 1.028703311283776507E-14, 37.00000000000000711, 83.99999999999998579 ) ) ;
#11710=VECTOR ( 'NONE', #10549, 1000.000000000000000 ) ;
#11719=FACE_OUTER_BOUND ( 'NONE', #9091, .T. ) ;
#11721=CARTESIAN_POINT ( 'NONE',  ( -54.52327687265815825, 0.000000000000000000, -111.3697098814011923 ) ) ;
#11725=DIRECTION ( 'NONE',  ( 0.000000000000000000, 0.000000000000000000, -1.000000000000000000 ) ) ;
#11745=EDGE_CURVE ( 'NONE', #15608, #5658, #18138, .T. ) ;
#11746=CARTESIAN_POINT ( 'NONE',  ( 0.000000000000000000, 25.00000000000000000, 0.000000000000000000 ) ) ;
#11767=TOROIDAL_SURFACE ( 'NONE', #14721, 8.000000000000014211, 2.000000000000000000 ) ;
#11791=LINE ( 'NONE', #15476, #36 ) ;
#11795=VERTEX_POINT ( 'NONE', #4042 ) ;
#11817=EDGE_CURVE ( 'NONE', #14037, #17029, #15959, .T. ) ;
#11829=DIRECTION ( 'NONE',  ( -0.000000000000000000, -1.000000000000000000, -0.000000000000000000 ) ) ;
#11844=TOROIDAL_SURFACE ( 'NONE', #11099, 8.000000000000014211, 2.000000000000000000 ) ;
#11884=AXIS2_PLACEMENT_3D ( 'NONE', #12548, #5293, #19312 ) ;
#11886=ADVANCED_FACE ( 'NONE', ( #18259 ), #19517, .T. ) ;
#11887=EDGE_CURVE ( 'NONE', #19122, #3529, #2683, .T. ) ;
#11894=ADVANCED_FACE ( 'NONE', ( #18044 ), #7459, .T. ) ;
#11900=VECTOR ( 'NONE', #3432, 1000.000000000000000 ) ;
#11905=DIRECTION ( 'NONE',  ( 0.000000000000000000, 0.000000000000000000, 1.000000000000000000 ) ) ;
#11907=LINE ( 'NONE', #3153, #20933 ) ;
#11910=EDGE_CURVE ( 'NONE', #1991, #1532, #6754, .T. ) ;
#11917=VERTEX_POINT ( 'NONE', #803 ) ;
#11928=VECTOR ( 'NONE', #17966, 1000.000000000000000 ) ;
#11941=CIRCLE ( 'NONE', #14149, 124.0000000000000000 ) ;
#11944=CARTESIAN_POINT ( 'NONE',  ( -164.0000000000000000, 18.00000000000000355, -7.999999999999979572 ) ) ;
#11951=DIRECTION ( 'NONE',  ( 0.000000000000000000, 0.000000000000000000, 1.000000000000000000 ) ) ;
#11955=AXIS2_PLACEMENT_3D ( 'NONE', #3908, #7355, #4247 ) ;
#11970=EDGE_CURVE ( 'NONE', #18877, #9038, #12657, .T. ) ;
#11996=CARTESIAN_POINT ( 'NONE',  ( -164.0000000000000000, 1.999999999999998224, 53.76161406891260697 ) ) ;
#12001=CYLINDRICAL_SURFACE ( 'NONE', #5436, 120.0000000000000000 ) ;
#12002=CARTESIAN_POINT ( 'NONE',  ( -55.40268456415264353, 18.00000000000000355, -113.1659955246495883 ) ) ;
#12005=DIRECTION ( 'NONE',  ( 0.8981428216242005602, -3.051058334780146661E-15, -0.4397038457472480788 ) ) ;
#12008=DIRECTION ( 'NONE',  ( 0.000000000000000000, 0.000000000000000000, 1.000000000000000000 ) ) ;
#12032=ADVANCED_FACE ( 'NONE', ( #9645 ), #4663, .F. ) ;
#12035=CARTESIAN_POINT ( 'NONE',  ( -164.0000000000000000, 18.00000000000000355, 53.76161406891260697 ) ) ;
#12049=CARTESIAN_POINT ( 'NONE',  ( -164.0000000000000000, 18.00000000000000355, 4.016841501203319170E-14 ) ) ;
#12062=ORIENTED_EDGE ( 'NONE', *, *, #20170, .F. ) ;
#12069=DIRECTION ( 'NONE',  ( 0.000000000000000000, 0.000000000000000000, 1.000000000000000000 ) ) ;
#12108=CARTESIAN_POINT ( 'NONE',  ( -157.5176307659779127, 0.000000000000000000, 60.94675664190624786 ) ) ;
#12119=CARTESIAN_POINT ( 'NONE',  ( -146.5000000000000000, 20.00000000000000000, 2.081668171172168513E-14 ) ) ;
#12122=FACE_OUTER_BOUND ( 'NONE', #6818, .T. ) ;
#12125=CIRCLE ( 'NONE', #2207, 2.000000000000000000 ) ;
#12151=CARTESIAN_POINT ( 'NONE',  ( 54.52327687265660927, 0.000000000000000000, 111.3697098814019029 ) ) ;
#12156=AXIS2_PLACEMENT_3D ( 'NONE', #8682, #15731, #5240 ) ;
#12157=VERTEX_POINT ( 'NONE', #12035 ) ;
#12168=CARTESIAN_POINT ( 'NONE',  ( 54.52327687265662348, 0.000000000000000000, -111.3697098814019313 ) ) ;
#12172=LINE ( 'NONE', #15740, #15816 ) ;
#12193=ADVANCED_FACE ( 'NONE', ( #18918 ), #10440, .T. ) ;
#12196=LINE ( 'NONE', #4934, #18177 ) ;
#12209=ORIENTED_EDGE ( 'NONE', *, *, #15684, .F. ) ;
#12211=( BOUNDED_CURVE ( )  B_SPLINE_CURVE ( 3, ( #9299, #7578, #19847, #7466 ),
 .UNSPECIFIED., .F., .T. ) 
 B_SPLINE_CURVE_WITH_KNOTS ( ( 4, 4 ),
 ( 0.000000000000000000, 1.570796326794896558 ),
 .UNSPECIFIED. ) 
 CURVE ( )  GEOMETRIC_REPRESENTATION_ITEM ( )  RATIONAL_B_SPLINE_CURVE ( ( 1.000000000000000000, 0.8047378541243649375, 0.8047378541243649375, 1.000000000000000000 ) ) 
 REPRESENTATION_ITEM ( '' )  );
#12301=CARTESIAN_POINT ( 'NONE',  ( -157.5176307659779411, 0.000000000000000000, -60.94675664190620523 ) ) ;
#12304=LINE ( 'NONE', #22583, #16029 ) ;
#12310=CARTESIAN_POINT ( 'NONE',  ( 158.3970384574715808, 18.00000000000000355, -62.74304228515678261 ) ) ;
#12333=EDGE_CURVE ( 'NONE', #9403, #20163, #4856, .T. ) ;
#12348=CARTESIAN_POINT ( 'NONE',  ( 163.9999999999998863, 20.00000000000000000, 8.000000000002229328 ) ) ;
#12355=CARTESIAN_POINT ( 'NONE',  ( -146.5000000000000000, 20.00000000000000000, -9.999999999999980460 ) ) ;
#12358=FACE_OUTER_BOUND ( 'NONE', #6070, .T. ) ;
#12375=EDGE_CURVE ( 'NONE', #18579, #4119, #11334, .T. ) ;
#12403=CARTESIAN_POINT ( 'NONE',  ( 1.458023040593673859E-15, 0.000000000000000000, 9.999999999999994671 ) ) ;
#12423=EDGE_CURVE ( 'NONE', #19859, #979, #20995, .T. ) ;
#12435=DIRECTION ( 'NONE',  ( 0.000000000000000000, 0.000000000000000000, 1.000000000000000000 ) ) ;
#12445=DIRECTION ( 'NONE',  ( -1.396592535537253658E-14, 0.000000000000000000, -1.000000000000000000 ) ) ;
#12448=VECTOR ( 'NONE', #10419, 1000.000000000000000 ) ;
#12456=DIRECTION ( 'NONE',  ( -1.387778780781445676E-14, 0.000000000000000000, -1.000000000000000000 ) ) ;
#12461=AXIS2_PLACEMENT_3D ( 'NONE', #1154, #4342, #2645 ) ;
#12464=DIRECTION ( 'NONE',  ( -0.000000000000000000, -1.000000000000000000, -0.000000000000000000 ) ) ;
#12470=EDGE_CURVE ( 'NONE', #19122, #11172, #19433, .T. ) ;
#12477=CIRCLE ( 'NONE', #8419, 8.000000000000014211 ) ;
#12489=CARTESIAN_POINT ( 'NONE',  ( 163.9999999999998863, 1.999999999999998224, 8.000000000002229328 ) ) ;
#12503=FACE_BOUND ( 'NONE', #10012, .T. ) ;
#12514=DIRECTION ( 'NONE',  ( 1.000000000000000000, -0.000000000000000000, -1.458023040593674599E-16 ) ) ;
#12535=VECTOR ( 'NONE', #16032, 1000.000000000000114 ) ;
#12540=AXIS2_PLACEMENT_3D ( 'NONE', #19741, #18505, #7820 ) ;
#12548=CARTESIAN_POINT ( 'NONE',  ( 0.000000000000000000, 37.00000000000000711, 0.000000000000000000 ) ) ;
#12557=AXIS2_PLACEMENT_3D ( 'NONE', #17105, #1367, #8344 ) ;
#12561=DIRECTION ( 'NONE',  ( 0.8981428216242033358, -0.000000000000000000, 0.4397038457472425277 ) ) ;
#12577=FACE_OUTER_BOUND ( 'NONE', #12976, .T. ) ;
#12589=PLANE ( 'NONE',  #9169 ) ;
#12609=ORIENTED_EDGE ( 'NONE', *, *, #14925, .F. ) ;
#12621=ORIENTED_EDGE ( 'NONE', *, *, #22387, .T. ) ;
#12635=ADVANCED_FACE ( 'NONE', ( #4258 ), #9202, .T. ) ;
#12637=CARTESIAN_POINT ( 'NONE',  ( -162.0000000000000000, 1.999999999999998224, 53.76161406891260697 ) ) ;
#12647=EDGE_LOOP ( 'NONE', ( #14802, #3835, #9206, #21142, #13479 ) ) ;
#12650=DIRECTION ( 'NONE',  ( 0.000000000000000000, 0.000000000000000000, -1.000000000000000000 ) ) ;
#12655=EDGE_CURVE ( 'NONE', #22152, #10082, #18805, .T. ) ;
#12657=CIRCLE ( 'NONE', #2003, 10.00000000000000888 ) ;
#12684=CARTESIAN_POINT ( 'NONE',  ( 161.9999999999998579, 20.00000000000000000, -10.00000000000224176 ) ) ;
#12690=VECTOR ( 'NONE', #4568, 1000.000000000000000 ) ;
#12730=ADVANCED_FACE ( 'NONE', ( #4933 ), #16914, .F. ) ;
#12743=ADVANCED_FACE ( 'NONE', ( #18727 ), #13363, .T. ) ;
#12752=DIRECTION ( 'NONE',  ( 0.000000000000000000, -1.000000000000000000, -0.000000000000000000 ) ) ;
#12753=DIRECTION ( 'NONE',  ( 0.000000000000000000, -0.000000000000000000, 1.000000000000000000 ) ) ;
#12768=CYLINDRICAL_SURFACE ( 'NONE', #11439, 2.000000000000004441 ) ;
#12769=CARTESIAN_POINT ( 'NONE',  ( -90.00000000000000000, 0.000000000000000000, 10.99999999999999289 ) ) ;
#12788=ORIENTED_EDGE ( 'NONE', *, *, #13051, .T. ) ;
#12800=AXIS2_PLACEMENT_3D ( 'NONE', #11210, #5908, #14906 ) ;
#12801=CARTESIAN_POINT ( 'NONE',  ( 0.000000000000000000, 23.00000000000000000, 0.000000000000000000 ) ) ;
#12804=CARTESIAN_POINT ( 'NONE',  ( 146.4999999999998579, 18.00000000000000355, 10.00000000000198952 ) ) ;
#12807=CARTESIAN_POINT ( 'NONE',  ( -146.5000000000000000, 1.999999999999998224, -9.999999999999980460 ) ) ;
#12808=CARTESIAN_POINT ( 'NONE',  ( 55.40268456415110165, 20.00000000000000000, 113.1659955246503415 ) ) ;
#12832=AXIS2_PLACEMENT_3D ( 'NONE', #3152, #4866, #10166 ) ;
#12838=ORIENTED_EDGE ( 'NONE', *, *, #22653, .F. ) ;
#12841=DIRECTION ( 'NONE',  ( 0.000000000000000000, -1.000000000000000000, -0.000000000000000000 ) ) ;
#12844=EDGE_LOOP ( 'NONE', ( #14532, #4760 ) ) ;
#12848=VECTOR ( 'NONE', #1052, 1000.000000000000000 ) ;
#12850=ADVANCED_FACE ( 'NONE', ( #15881, #127 ), #3450, .F. ) ;
#12861=CARTESIAN_POINT ( 'NONE',  ( -162.0000000000000000, 0.000000000000000000, -9.999999999999978684 ) ) ;
#12878=ADVANCED_FACE ( 'NONE', ( #1730 ), #19176, .T. ) ;
#12880=ADVANCED_FACE ( 'NONE', ( #7231 ), #8191, .T. ) ;
#12881=CARTESIAN_POINT ( 'NONE',  ( 146.4999999999998863, 1.999999999999998224, 8.000000000001989520 ) ) ;
#12897=EDGE_LOOP ( 'NONE', ( #20388, #4818, #39, #16917 ) ) ;
#12908=FACE_OUTER_BOUND ( 'NONE', #20421, .T. ) ;
#12914=DIRECTION ( 'NONE',  ( 0.000000000000000000, 0.000000000000000000, 1.000000000000000000 ) ) ;
#12941=CYLINDRICAL_SURFACE ( 'NONE', #6280, 78.99999999999998579 ) ;
#12963=DIRECTION ( 'NONE',  ( -0.8981428216242030027, 0.000000000000000000, -0.4397038457472430273 ) ) ;
#12964=DIRECTION ( 'NONE',  ( -0.000000000000000000, -1.000000000000000000, -0.000000000000000000 ) ) ;
#12976=EDGE_LOOP ( 'NONE', ( #1831, #22487, #15394, #2153 ) ) ;
#12978=CIRCLE ( 'NONE', #3048, 117.0000000000000000 ) ;
#12980=FACE_OUTER_BOUND ( 'NONE', #5218, .T. ) ;
#12982=CARTESIAN_POINT ( 'NONE',  ( 55.40268456415107323, 1.999999999999998224, -113.1659955246503557 ) ) ;
#12984=EDGE_LOOP ( 'NONE', ( #3217, #15969, #6183, #10158 ) ) ;
#12992=DIRECTION ( 'NONE',  ( 0.000000000000000000, 0.000000000000000000, 1.000000000000000000 ) ) ;
#12998=DIRECTION ( 'NONE',  ( 0.000000000000000000, 0.000000000000000000, 1.000000000000000000 ) ) ;
#13002=CIRCLE ( 'NONE', #15943, 120.0000000000000000 ) ;
#13028=CARTESIAN_POINT ( 'NONE',  ( -90.00000000000000000, 45.00100000000000477, 8.394090934816448357E-16 ) ) ;
#13030=FACE_OUTER_BOUND ( 'NONE', #6908, .T. ) ;
#13031=ORIENTED_EDGE ( 'NONE', *, *, #7815, .F. ) ;
#13035=DIRECTION ( 'NONE',  ( 0.000000000000000000, 0.000000000000000000, 1.000000000000000000 ) ) ;
#13051=EDGE_CURVE ( 'NONE', #2469, #10602, #4499, .T. ) ;
#13072=ADVANCED_FACE ( 'NONE', ( #17895 ), #1693, .F. ) ;
#13083=ORIENTED_EDGE ( 'NONE', *, *, #5387, .F. ) ;
#13093=CARTESIAN_POINT ( 'NONE',  ( 146.5000000000000000, 20.00000000000000000, -2.025191382850354537E-12 ) ) ;
#13105=CARTESIAN_POINT ( 'NONE',  ( -157.5176307659779411, 20.00000000000000000, -60.94675664190619813 ) ) ;
#13108=CARTESIAN_POINT ( 'NONE',  ( -1.109343863968193944E-13, 18.00000000000000355, -7.999999999999994671 ) ) ;
#13128=VECTOR ( 'NONE', #1536, 1000.000000000000114 ) ;
#13129=ORIENTED_EDGE ( 'NONE', *, *, #9657, .T. ) ;
#13144=CARTESIAN_POINT ( 'NONE',  ( 153.9999999999992610, 20.00000000000000000, 53.76161406891468175 ) ) ;
#13163=ORIENTED_EDGE ( 'NONE', *, *, #7445, .T. ) ;
#13167=EDGE_CURVE ( 'NONE', #5531, #1407, #20835, .T. ) ;
#13173=DIRECTION ( 'NONE',  ( -1.000000000000000000, 0.000000000000000000, 1.386679829960243376E-14 ) ) ;
#13174=DIRECTION ( 'NONE',  ( -0.000000000000000000, -1.000000000000000000, -0.000000000000000000 ) ) ;
#13180=EDGE_CURVE ( 'NONE', #7438, #10504, #21403, .T. ) ;
#13187=DIRECTION ( 'NONE',  ( 0.000000000000000000, 0.000000000000000000, 1.000000000000000000 ) ) ;
#13192=DIRECTION ( 'NONE',  ( -9.912705577010318154E-17, 0.000000000000000000, -1.000000000000000000 ) ) ;
#13223=AXIS2_PLACEMENT_3D ( 'NONE', #15729, #11829, #3178 ) ;
#13232=VECTOR ( 'NONE', #4512, 1000.000000000000000 ) ;
#13238=DIRECTION ( 'NONE',  ( 0.000000000000000000, 1.000000000000000000, -0.000000000000000000 ) ) ;
#13241=DIRECTION ( 'NONE',  ( -0.000000000000000000, -1.000000000000000000, -0.000000000000000000 ) ) ;
#13248=EDGE_LOOP ( 'NONE', ( #9753, #21822, #1604, #18026 ) ) ;
#13258=AXIS2_PLACEMENT_3D ( 'NONE', #17557, #2261, #1809 ) ;
#13259=DIRECTION ( 'NONE',  ( 0.000000000000000000, 0.000000000000000000, -1.000000000000000000 ) ) ;
#13271=AXIS2_PLACEMENT_3D ( 'NONE', #15372, #20626, #6612 ) ;
#13276=CIRCLE ( 'NONE', #3350, 2.000000000000001776 ) ;
#13278=ORIENTED_EDGE ( 'NONE', *, *, #11817, .T. ) ;
#13294=CARTESIAN_POINT ( 'NONE',  ( 0.000000000000000000, 25.00000000000000000, 0.000000000000000000 ) ) ;
#13295=CIRCLE ( 'NONE', #3368, 2.000000000000001776 ) ;
#13299=ORIENTED_EDGE ( 'NONE', *, *, #8342, .T. ) ;
#13300=DIRECTION ( 'NONE',  ( 0.000000000000000000, 0.000000000000000000, -1.000000000000000000 ) ) ;
#13304=EDGE_CURVE ( 'NONE', #14680, #7464, #5242, .T. ) ;
#13319=CARTESIAN_POINT ( 'NONE',  ( 163.9999999999998863, 20.00000000000000000, -8.000000000002268408 ) ) ;
#13327=EDGE_CURVE ( 'NONE', #16446, #7377, #16671, .T. ) ;
#13330=ORIENTED_EDGE ( 'NONE', *, *, #6496, .T. ) ;
#13345=DIRECTION ( 'NONE',  ( 0.000000000000000000, 0.000000000000000000, -1.000000000000000000 ) ) ;
#13352=TOROIDAL_SURFACE ( 'NONE', #161, 124.0000000000000000, 2.000000000000000000 ) ;
#13360=CARTESIAN_POINT ( 'NONE',  ( -1.089749515181836320E-13, 18.00000000000000355, 7.999999999999994671 ) ) ;
#13363=CYLINDRICAL_SURFACE ( 'NONE', #18111, 2.000000000000001776 ) ;
#13367=DIRECTION ( 'NONE',  ( -0.000000000000000000, -0.000000000000000000, -1.000000000000000000 ) ) ;
#13370=ORIENTED_EDGE ( 'NONE', *, *, #20170, .T. ) ;
#13376=ORIENTED_EDGE ( 'NONE', *, *, #6650, .T. ) ;
#13378=DIRECTION ( 'NONE',  ( 0.000000000000000000, -1.000000000000000000, 0.000000000000000000 ) ) ;
#13379=CIRCLE ( 'NONE', #6400, 2.000000000000001332 ) ;
#13384=ADVANCED_FACE ( 'NONE', ( #14084 ), #1554, .F. ) ;
#13390=TOROIDAL_SURFACE ( 'NONE', #13738, 8.000000000000014211, 2.000000000000000000 ) ;
#13404=TOROIDAL_SURFACE ( 'NONE', #4205, 10.00000000000000355, 2.000000000000000000 ) ;
#13417=CYLINDRICAL_SURFACE ( 'NONE', #14357, 83.99999999999998579 ) ;
#13433=ADVANCED_FACE ( 'NONE', ( #12358 ), #17765, .F. ) ;
#13437=CARTESIAN_POINT ( 'NONE',  ( 0.000000000000000000, 37.00000000000000711, 0.000000000000000000 ) ) ;
#13445=EDGE_CURVE ( 'NONE', #5068, #16242, #8928, .T. ) ;
#13471=DIRECTION ( 'NONE',  ( -1.000000000000000000, 0.000000000000000000, -1.372099599554301422E-14 ) ) ;
#13479=ORIENTED_EDGE ( 'NONE', *, *, #22366, .F. ) ;
#13494=CARTESIAN_POINT ( 'NONE',  ( 146.4999999999998579, 2.000000000000000000, 9.999999999997978506 ) ) ;
#13520=CARTESIAN_POINT ( 'NONE',  ( 0.000000000000000000, 23.00000000000000000, 118.0000000000000000 ) ) ;
#13524=CARTESIAN_POINT ( 'NONE',  ( -55.40268456415262932, 18.00000000000000355, 113.1659955246495883 ) ) ;
#13526=FACE_OUTER_BOUND ( 'NONE', #3772, .T. ) ;
#13528=ORIENTED_EDGE ( 'NONE', *, *, #4413, .F. ) ;
#13543=DIRECTION ( 'NONE',  ( 0.000000000000000000, -0.000000000000000000, 1.000000000000000000 ) ) ;
#13550=DIRECTION ( 'NONE',  ( -1.000000000000000000, 0.000000000000000000, 9.912705577010318154E-17 ) ) ;
#13555=CARTESIAN_POINT ( 'NONE',  ( -154.0000000000000000, 20.00000000000000000, 53.76161406891259986 ) ) ;
#13567=ADVANCED_FACE ( 'NONE', ( #6687 ), #10032, .T. ) ;
#13569=CARTESIAN_POINT ( 'NONE',  ( 0.000000000000000000, 25.00000000000000000, 0.000000000000000000 ) ) ;
#13572=AXIS2_PLACEMENT_3D ( 'NONE', #17384, #8321, #13300 ) ;
#13576=EDGE_LOOP ( 'NONE', ( #4805, #7182, #11164, #6489 ) ) ;
#13587=DIRECTION ( 'NONE',  ( 0.000000000000000000, 0.000000000000000000, -1.000000000000000000 ) ) ;
#13619=ORIENTED_EDGE ( 'NONE', *, *, #3011, .T. ) ;
#13622=AXIS2_PLACEMENT_3D ( 'NONE', #9325, #8257, #13543 ) ;
#13643=ORIENTED_EDGE ( 'NONE', *, *, #11970, .T. ) ;
#13645=ADVANCED_FACE ( 'NONE', ( #2798 ), #13352, .T. ) ;
#13647=PLANE ( 'NONE',  #14412 ) ;
#13651=ORIENTED_EDGE ( 'NONE', *, *, #2069, .F. ) ;
#13658=EDGE_CURVE ( 'NONE', #7377, #9416, #2707, .T. ) ;
#13679=DIRECTION ( 'NONE',  ( -0.000000000000000000, -1.000000000000000000, 0.000000000000000000 ) ) ;
#13683=CARTESIAN_POINT ( 'NONE',  ( -90.00000000000000000, 29.00000000000000355, 8.394090934816448357E-16 ) ) ;
#13693=LINE ( 'NONE', #22039, #9544 ) ;
#13695=AXIS2_PLACEMENT_3D ( 'NONE', #8046, #1055, #1180 ) ;
#13697=CARTESIAN_POINT ( 'NONE',  ( -164.0000000000000000, 20.00000000000000000, 10.00000000000001954 ) ) ;
#13729=ORIENTED_EDGE ( 'NONE', *, *, #17520, .F. ) ;
#13736=DIRECTION ( 'NONE',  ( 1.000000000000000000, 0.000000000000000000, 1.362186893977296347E-14 ) ) ;
#13738=AXIS2_PLACEMENT_3D ( 'NONE', #19020, #1044, #16903 ) ;
#13748=FACE_OUTER_BOUND ( 'NONE', #20393, .T. ) ;
#13750=AXIS2_PLACEMENT_3D ( 'NONE', #16667, #8254, #8140 ) ;
#13774=DIRECTION ( 'NONE',  ( 0.000000000000000000, -1.000000000000000000, 0.000000000000000000 ) ) ;
#13777=DIRECTION ( 'NONE',  ( 0.8981428216242087759, 0.000000000000000000, 0.4397038457472314255 ) ) ;
#13779=LINE ( 'NONE', #12049, #11710 ) ;
#13783=ORIENTED_EDGE ( 'NONE', *, *, #20623, .F. ) ;
#13836=ORIENTED_EDGE ( 'NONE', *, *, #16525, .T. ) ;
#13837=UNCERTAINTY_MEASURE_WITH_UNIT (LENGTH_MEASURE( 1.000000000000000082E-05 ), #17274, 'distance_accuracy_value', 'NONE');
#13840=EDGE_LOOP ( 'NONE', ( #2106, #11107, #6153, #15418 ) ) ;
#13841=DIRECTION ( 'NONE',  ( 0.000000000000000000, 0.000000000000000000, -1.000000000000000000 ) ) ;
#13857=CARTESIAN_POINT ( 'NONE',  ( -1.432836755002403442E-14, 25.00000000000000000, -117.0000000000000000 ) ) ;
#13866=ORIENTED_EDGE ( 'NONE', *, *, #18951, .T. ) ;
#13867=DIRECTION ( 'NONE',  ( 0.8981428216242088869, 0.000000000000000000, 0.4397038457472307593 ) ) ;
#13874=ADVANCED_FACE ( 'NONE', ( #17548 ), #7476, .T. ) ;
#13879=DIRECTION ( 'NONE',  ( 0.000000000000000000, 1.000000000000000000, -0.000000000000000000 ) ) ;
#13882=AXIS2_PLACEMENT_3D ( 'NONE', #688, #9167, #2293 ) ;
#13883=CARTESIAN_POINT ( 'NONE',  ( 55.40268456415108744, 18.00000000000000355, 113.1659955246503557 ) ) ;
#13888=EDGE_CURVE ( 'NONE', #2665, #1225, #8222, .T. ) ;
#13891=CYLINDRICAL_SURFACE ( 'NONE', #20620, 10.00000000000000888 ) ;
#13900=ORIENTED_EDGE ( 'NONE', *, *, #9966, .F. ) ;
#13906=DIRECTION ( 'NONE',  ( 0.000000000000000000, 1.000000000000000000, -0.000000000000000000 ) ) ;
#13921=CARTESIAN_POINT ( 'NONE',  ( -146.5000000000000000, 18.00000000000000355, -7.999999999999981348 ) ) ;
#13938=DIRECTION ( 'NONE',  ( 0.000000000000000000, -1.000000000000000000, 0.000000000000000000 ) ) ;
#13940=DIRECTION ( 'NONE',  ( -0.000000000000000000, -1.000000000000000000, -0.000000000000000000 ) ) ;
#13991=EDGE_CURVE ( 'NONE', #3529, #11795, #19070, .T. ) ;
#14001=CIRCLE ( 'NONE', #19471, 124.0000000000000000 ) ;
#14005=CARTESIAN_POINT ( 'NONE',  ( 163.9999999999992610, 1.999999999999998224, -53.76161406891485228 ) ) ;
#14021=DIRECTION ( 'NONE',  ( -0.000000000000000000, -1.000000000000000000, 0.000000000000000000 ) ) ;
#14037=VERTEX_POINT ( 'NONE', #15097 ) ;
#14045=VERTEX_POINT ( 'NONE', #1192 ) ;
#14047=EDGE_LOOP ( 'NONE', ( #22100, #3128, #9702, #20306, #7068 ) ) ;
#14055=CARTESIAN_POINT ( 'NONE',  ( -164.0000000000000000, 2.000000000000000000, -7.999999999999979572 ) ) ;
#14065=CARTESIAN_POINT ( 'NONE',  ( -162.0000000000000000, 0.000000000000000000, -53.76161406891256433 ) ) ;
#14077=ORIENTED_EDGE ( 'NONE', *, *, #19865, .T. ) ;
#14084=FACE_OUTER_BOUND ( 'NONE', #16564, .T. ) ;
#14091=AXIS2_PLACEMENT_3D ( 'NONE', #5684, #18127, #14565 ) ;
#14097=VECTOR ( 'NONE', #259, 1000.000000000000000 ) ;
#14125=ORIENTED_EDGE ( 'NONE', *, *, #20279, .F. ) ;
#14135=EDGE_CURVE ( 'NONE', #7464, #6252, #19297, .T. ) ;
#14148=DIRECTION ( 'NONE',  ( -0.4397038457472313144, 0.000000000000000000, -0.8981428216242086648 ) ) ;
#14149=AXIS2_PLACEMENT_3D ( 'NONE', #18521, #955, #4366 ) ;
#14158=ORIENTED_EDGE ( 'NONE', *, *, #17570, .F. ) ;
#14166=ORIENTED_EDGE ( 'NONE', *, *, #14591, .T. ) ;
#14184=DIRECTION ( 'NONE',  ( 2.449293598294706414E-16, 0.000000000000000000, 1.000000000000000000 ) ) ;
#14198=DIRECTION ( 'NONE',  ( -0.4397038457472354778, 0.000000000000000000, -0.8981428216242066664 ) ) ;
#14210=EDGE_CURVE ( 'NONE', #5236, #6260, #21779, .T. ) ;
#14221=DIRECTION ( 'NONE',  ( 1.000000000000000000, -0.000000000000000000, 0.000000000000000000 ) ) ;
#14242=DIRECTION ( 'NONE',  ( -0.000000000000000000, -1.000000000000000000, -0.000000000000000000 ) ) ;
#14248=TOROIDAL_SURFACE ( 'NONE', #4315, 124.0000000000000000, 2.000000000000000000 ) ;
#14258=CIRCLE ( 'NONE', #13882, 2.000000000000007550 ) ;
#14269=ORIENTED_EDGE ( 'NONE', *, *, #2892, .F. ) ;
#14270=CARTESIAN_POINT ( 'NONE',  ( 163.9999999999992610, 18.00000000000000355, 53.76161406891480965 ) ) ;
#14278=FACE_OUTER_BOUND ( 'NONE', #18931, .T. ) ;
#14284=VECTOR ( 'NONE', #1808, 1000.000000000000000 ) ;
#14293=ORIENTED_EDGE ( 'NONE', *, *, #20841, .F. ) ;
#14315=ORIENTED_EDGE ( 'NONE', *, *, #4672, .T. ) ;
#14321=CIRCLE ( 'NONE', #19057, 2.000000000000001332 ) ;
#14340=CARTESIAN_POINT ( 'NONE',  ( -162.0000000000000000, 2.000000000000000000, 0.000000000000000000 ) ) ;
#14352=EDGE_LOOP ( 'NONE', ( #13528, #5598, #7044, #11125, #18947 ) ) ;
#14357=AXIS2_PLACEMENT_3D ( 'NONE', #22314, #17183, #22211 ) ;
#14358=AXIS2_PLACEMENT_3D ( 'NONE', #16255, #18191, #14527 ) ;
#14397=ORIENTED_EDGE ( 'NONE', *, *, #19865, .F. ) ;
#14403=DIRECTION ( 'NONE',  ( -1.386679829960243061E-14, 0.000000000000000000, -1.000000000000000000 ) ) ;
#14412=AXIS2_PLACEMENT_3D ( 'NONE', #2736, #4765, #20396 ) ;
#14437=DIRECTION ( 'NONE',  ( -1.387778780781445676E-14, 0.000000000000000000, 1.000000000000000000 ) ) ;
#14460=CARTESIAN_POINT ( 'NONE',  ( -164.0000000000000000, 1.999999999999998224, 53.76161406891260697 ) ) ;
#14466=EDGE_CURVE ( 'NONE', #15997, #2837, #22524, .T. ) ;
#14508=CARTESIAN_POINT ( 'NONE',  ( -146.5000000000000000, 1.999999999999998224, 2.081668171172168513E-14 ) ) ;
#14514=VERTEX_POINT ( 'NONE', #5080 ) ;
#14524=FACE_BOUND ( 'NONE', #118, .T. ) ;
#14527=DIRECTION ( 'NONE',  ( 0.000000000000000000, 0.000000000000000000, -1.000000000000000000 ) ) ;
#14531=FACE_OUTER_BOUND ( 'NONE', #11601, .T. ) ;
#14532=ORIENTED_EDGE ( 'NONE', *, *, #15684, .T. ) ;
#14555=ADVANCED_FACE ( 'NONE', ( #6922 ), #11661, .T. ) ;
#14565=DIRECTION ( 'NONE',  ( 0.000000000000000000, 0.000000000000000000, 1.000000000000000000 ) ) ;
#14567=CARTESIAN_POINT ( 'NONE',  ( 163.9999999999998863, 0.8284271247461897358, 8.000000000002229328 ) ) ;
#14578=CARTESIAN_POINT ( 'NONE',  ( -162.0000000000000000, 20.00000000000000000, -9.999999999999978684 ) ) ;
#14581=PLANE ( 'NONE',  #8436 ) ;
#14585=EDGE_LOOP ( 'NONE', ( #21251, #15605 ) ) ;
#14591=EDGE_CURVE ( 'NONE', #10233, #21383, #4919, .T. ) ;
#14592=DIRECTION ( 'NONE',  ( -0.000000000000000000, -1.000000000000000000, -0.000000000000000000 ) ) ;
#14598=EDGE_LOOP ( 'NONE', ( #21300, #7949, #14166, #10170 ) ) ;
#14618=DIRECTION ( 'NONE',  ( 1.000000000000000000, -0.000000000000000000, -9.912705577010318154E-17 ) ) ;
#14647=ORIENTED_EDGE ( 'NONE', *, *, #11319, .T. ) ;
#14657=ADVANCED_FACE ( 'NONE', ( #11493 ), #13404, .T. ) ;
#14677=LINE ( 'NONE', #11102, #6689 ) ;
#14680=VERTEX_POINT ( 'NONE', #7919 ) ;
#14684=TOROIDAL_SURFACE ( 'NONE', #21600, 8.000000000000014211, 2.000000000000000000 ) ;
#14703=EDGE_CURVE ( 'NONE', #1627, #3659, #190, .T. ) ;
#14710=EDGE_LOOP ( 'NONE', ( #15868, #14933, #2389, #18769 ) ) ;
#14715=CARTESIAN_POINT ( 'NONE',  ( 0.000000000000000000, 1.999999999999998224, 0.000000000000000000 ) ) ;
#14719=CARTESIAN_POINT ( 'NONE',  ( 162.0000000000000000, 0.000000000000000000, 2.222801351277976832E-12 ) ) ;
#14721=AXIS2_PLACEMENT_3D ( 'NONE', #7840, #9204, #13035 ) ;
#14734=ORIENTED_EDGE ( 'NONE', *, *, #2794, .T. ) ;
#14738=ORIENTED_EDGE ( 'NONE', *, *, #13051, .F. ) ;
#14743=DIRECTION ( 'NONE',  ( 0.000000000000000000, 0.000000000000000000, 1.000000000000000000 ) ) ;
#14757=FACE_OUTER_BOUND ( 'NONE', #1742, .T. ) ;
#14773=VECTOR ( 'NONE', #18367, 1000.000000000000000 ) ;
#14786=FACE_OUTER_BOUND ( 'NONE', #10838, .T. ) ;
#14792=VECTOR ( 'NONE', #14242, 1000.000000000000000 ) ;
#14802=ORIENTED_EDGE ( 'NONE', *, *, #8342, .F. ) ;
#14830=DIRECTION ( 'NONE',  ( 0.000000000000000000, 0.000000000000000000, 1.000000000000000000 ) ) ;
#14865=DIRECTION ( 'NONE',  ( -1.000000000000000000, 0.000000000000000000, -1.387778780781444413E-14 ) ) ;
#14871=LINE ( 'NONE', #13697, #2412 ) ;
#14876=FACE_OUTER_BOUND ( 'NONE', #11149, .T. ) ;
#14906=DIRECTION ( 'NONE',  ( 0.000000000000000000, 0.000000000000000000, 1.000000000000000000 ) ) ;
#14925=EDGE_CURVE ( 'NONE', #1532, #2916, #15625, .T. ) ;
#14933=ORIENTED_EDGE ( 'NONE', *, *, #20150, .T. ) ;
#14937=DIRECTION ( 'NONE',  ( -0.8981428216242088869, 0.000000000000000000, -0.4397038457472307593 ) ) ;
#14943=ADVANCED_FACE ( 'NONE', ( #17343 ), #7412, .T. ) ;
#14956=DIRECTION ( 'NONE',  ( 0.000000000000000000, 0.000000000000000000, 1.000000000000000000 ) ) ;
#14959=DIRECTION ( 'NONE',  ( 9.912705577010319386E-17, 0.000000000000000000, 1.000000000000000000 ) ) ;
#14963=ORIENTED_EDGE ( 'NONE', *, *, #1776, .T. ) ;
#14997=EDGE_CURVE ( 'NONE', #7423, #15641, #10551, .T. ) ;
#14999=LINE ( 'NONE', #21732, #13232 ) ;
#15007=EDGE_LOOP ( 'NONE', ( #1545, #18047, #2874, #15643 ) ) ;
#15018=ORIENTED_EDGE ( 'NONE', *, *, #4338, .T. ) ;
#15023=DIRECTION ( 'NONE',  ( 1.396592535537253658E-14, -0.000000000000000000, 1.000000000000000000 ) ) ;
#15044=ADVANCED_FACE ( 'NONE', ( #12980 ), #18246, .T. ) ;
#15064=DIRECTION ( 'NONE',  ( 1.000000000000000000, 0.000000000000000000, -2.449293598294699019E-16 ) ) ;
#15072=DIRECTION ( 'NONE',  ( 0.000000000000000000, 0.000000000000000000, 1.000000000000000000 ) ) ;
#15079=DIRECTION ( 'NONE',  ( -0.000000000000000000, -1.000000000000000000, 0.000000000000000000 ) ) ;
#15085=PRESENTATION_STYLE_ASSIGNMENT (( #2992 ) ) ;
#15097=CARTESIAN_POINT ( 'NONE',  ( 55.40268456415108744, 1.999999999999998224, 113.1659955246503557 ) ) ;
#15101=CARTESIAN_POINT ( 'NONE',  ( -1.362186893977295590E-13, 18.00000000000000355, 9.999999999999994671 ) ) ;
#15112=CIRCLE ( 'NONE', #13271, 96.00000000000000000 ) ;
#15137=LINE ( 'NONE', #2925, #18123 ) ;
#15147=AXIS2_PLACEMENT_3D ( 'NONE', #17077, #1443, #1336 ) ;
#15148=AXIS2_PLACEMENT_3D ( 'NONE', #15978, #216, #7100 ) ;
#15150=EDGE_CURVE ( 'NONE', #6252, #3529, #18348, .T. ) ;
#15152=DIRECTION ( 'NONE',  ( -1.000000000000000000, 0.000000000000000000, 9.912705577010318154E-17 ) ) ;
#15168=DIRECTION ( 'NONE',  ( -0.8981428216242089979, 0.000000000000000000, -0.4397038457472307593 ) ) ;
#15174=CYLINDRICAL_SURFACE ( 'NONE', #16921, 126.0000000000000000 ) ;
#15175=EDGE_CURVE ( 'NONE', #8292, #1407, #21875, .T. ) ;
#15179=DIRECTION ( 'NONE',  ( -0.000000000000000000, -1.000000000000000000, -0.000000000000000000 ) ) ;
#15193=CARTESIAN_POINT ( 'NONE',  ( 146.5000000000000000, 0.000000000000000000, -2.025191382850354537E-12 ) ) ;
#15199=DIRECTION ( 'NONE',  ( 0.000000000000000000, 0.000000000000000000, 1.000000000000000000 ) ) ;
#15208=ADVANCED_FACE ( 'NONE', ( #6620 ), #13647, .T. ) ;
#15209=CIRCLE ( 'NONE', #9322, 2.000000000000001776 ) ;
#15219=VERTEX_POINT ( 'NONE', #4438 ) ;
#15227=DIRECTION ( 'NONE',  ( 0.000000000000000000, 1.000000000000000000, -0.000000000000000000 ) ) ;
#15249=CYLINDRICAL_SURFACE ( 'NONE', #20832, 2.000000000000001776 ) ;
#15255=ORIENTED_EDGE ( 'NONE', *, *, #9406, .F. ) ;
#15263=ORIENTED_EDGE ( 'NONE', *, *, #21858, .T. ) ;
#15271=AXIS2_PLACEMENT_3D ( 'NONE', #15882, #17365, #5272 ) ;
#15284=AXIS2_PLACEMENT_3D ( 'NONE', #18178, #364, #14743 ) ;
#15291=ADVANCED_FACE ( 'NONE', ( #22546, #21084 ), #20846, .T. ) ;
#15302=DIRECTION ( 'NONE',  ( 0.000000000000000000, 0.000000000000000000, 1.000000000000000000 ) ) ;
#15304=ORIENTED_EDGE ( 'NONE', *, *, #16967, .F. ) ;
#15308=DIRECTION ( 'NONE',  ( 0.8981428216242027807, -0.000000000000000000, -0.4397038457472431938 ) ) ;
#15353=CARTESIAN_POINT ( 'NONE',  ( -162.0000000000000000, 1.999999999999998224, 3.967855629237425111E-14 ) ) ;
#15372=CARTESIAN_POINT ( 'NONE',  ( 0.000000000000000000, 45.00000000000000711, 0.000000000000000000 ) ) ;
#15375=CIRCLE ( 'NONE', #5066, 120.0000000000000000 ) ;
#15394=ORIENTED_EDGE ( 'NONE', *, *, #16605, .F. ) ;
#15418=ORIENTED_EDGE ( 'NONE', *, *, #170, .F. ) ;
#15440=DIRECTION ( 'NONE',  ( -0.000000000000000000, -1.000000000000000000, -0.000000000000000000 ) ) ;
#15455=CARTESIAN_POINT ( 'NONE',  ( -146.5000000000000000, 20.00000000000000000, -9.999999999999980460 ) ) ;
#15457=CIRCLE ( 'NONE', #21628, 2.000000000000004441 ) ;
#15458=VECTOR ( 'NONE', #16139, 1000.000000000000000 ) ;
#15476=CARTESIAN_POINT ( 'NONE',  ( 0.000000000000000000, 0.000000000000000000, -101.0000000000000000 ) ) ;
#15490=ORIENTED_EDGE ( 'NONE', *, *, #11319, .F. ) ;
#15514=DIRECTION ( 'NONE',  ( 0.8981428216242088869, -0.000000000000000000, 0.4397038457472307593 ) ) ;
#15568=EDGE_CURVE ( 'NONE', #1627, #18838, #16030, .T. ) ;
#15582=CARTESIAN_POINT ( 'NONE',  ( 0.000000000000000000, 25.00000000000000000, 0.000000000000000000 ) ) ;
#15605=ORIENTED_EDGE ( 'NONE', *, *, #6496, .F. ) ;
#15608=VERTEX_POINT ( 'NONE', #6917 ) ;
#15625=LINE ( 'NONE', #10443, #5944 ) ;
#15641=VERTEX_POINT ( 'NONE', #20931 ) ;
#15643=ORIENTED_EDGE ( 'NONE', *, *, #16400, .F. ) ;
#15654=CARTESIAN_POINT ( 'NONE',  ( 0.000000000000000000, 37.00000000000000711, -101.0000000000000000 ) ) ;
#15661=CARTESIAN_POINT ( 'NONE',  ( 0.000000000000000000, 20.00000000000000000, -120.0000000000000000 ) ) ;
#15680=ORIENTED_EDGE ( 'NONE', *, *, #16427, .T. ) ;
#15681=ORIENTED_EDGE ( 'NONE', *, *, #11458, .T. ) ;
#15684=EDGE_CURVE ( 'NONE', #979, #9760, #5881, .T. ) ;
#15694=CARTESIAN_POINT ( 'NONE',  ( 153.9999999999992610, 1.999999999999998224, -53.76161406891471017 ) ) ;
#15704=ADVANCED_FACE ( 'NONE', ( #14757 ), #11767, .T. ) ;
#15713=DIRECTION ( 'NONE',  ( -0.000000000000000000, -1.000000000000000000, -0.000000000000000000 ) ) ;
#15729=CARTESIAN_POINT ( 'NONE',  ( 0.000000000000000000, 37.00000000000000711, 0.000000000000000000 ) ) ;
#15731=DIRECTION ( 'NONE',  ( -0.000000000000000000, -1.000000000000000000, -0.000000000000000000 ) ) ;
#15735=ADVANCED_FACE ( 'NONE', ( #12908 ), #7371, .T. ) ;
#15740=CARTESIAN_POINT ( 'NONE',  ( 158.3970384574715808, 20.00000000000000000, 62.74304228515676130 ) ) ;
#15751=ORIENTED_EDGE ( 'NONE', *, *, #16400, .T. ) ;
#15753=ORIENTED_EDGE ( 'NONE', *, *, #3283, .T. ) ;
#15759=CARTESIAN_POINT ( 'NONE',  ( 153.9999999999992610, 18.00000000000000355, -53.76161406891471017 ) ) ;
#15761=CIRCLE ( 'NONE', #10970, 83.99999999999998579 ) ;
#15767=EDGE_LOOP ( 'NONE', ( #17638, #8625 ) ) ;
#15773=VERTEX_POINT ( 'NONE', #1591 ) ;
#15775=CARTESIAN_POINT ( 'NONE',  ( 161.9999999999992610, 0.000000000000000000, -53.76161406891482386 ) ) ;
#15780=DIRECTION ( 'NONE',  ( 1.000000000000000000, 0.000000000000000000, -1.386679829960243376E-14 ) ) ;
#15782=ORIENTED_EDGE ( 'NONE', *, *, #13327, .F. ) ;
#15793=EDGE_CURVE ( 'NONE', #15219, #6576, #9730, .T. ) ;
#15804=LINE ( 'NONE', #12355, #3607 ) ;
#15809=DIRECTION ( 'NONE',  ( -0.8981428216242087759, 0.000000000000000000, 0.4397038457472309259 ) ) ;
#15816=VECTOR ( 'NONE', #17463, 1000.000000000000000 ) ;
#15819=CIRCLE ( 'NONE', #20172, 117.0000000000000000 ) ;
#15860=CARTESIAN_POINT ( 'NONE',  ( 0.000000000000000000, 20.00000000000000000, -126.0000000000000000 ) ) ;
#15868=ORIENTED_EDGE ( 'NONE', *, *, #20841, .T. ) ;
#15881=FACE_OUTER_BOUND ( 'NONE', #17612, .T. ) ;
#15882=CARTESIAN_POINT ( 'NONE',  ( 0.000000000000000000, 29.00000000000000355, 0.000000000000000000 ) ) ;
#15886=EDGE_CURVE ( 'NONE', #17969, #9954, #6994, .T. ) ;
#15916=LINE ( 'NONE', #16141, #9224 ) ;
#15919=ORIENTED_EDGE ( 'NONE', *, *, #15568, .T. ) ;
#15939=ORIENTED_EDGE ( 'NONE', *, *, #13304, .T. ) ;
#15942=VERTEX_POINT ( 'NONE', #10293 ) ;
#15943=AXIS2_PLACEMENT_3D ( 'NONE', #22403, #4956, #20809 ) ;
#15959=CIRCLE ( 'NONE', #18860, 2.000000000000004441 ) ;
#15967=CARTESIAN_POINT ( 'NONE',  ( -54.52327687265812983, 1.999999999999998224, 111.3697098814011923 ) ) ;
#15969=ORIENTED_EDGE ( 'NONE', *, *, #4169, .T. ) ;
#15975=EDGE_CURVE ( 'NONE', #16242, #5068, #15112, .T. ) ;
#15978=CARTESIAN_POINT ( 'NONE',  ( 0.000000000000000000, 1.999999999999998224, 0.000000000000000000 ) ) ;
#15979=EDGE_CURVE ( 'NONE', #10504, #19051, #6509, .T. ) ;
#15981=DIRECTION ( 'NONE',  ( 1.000000000000000000, 0.000000000000000000, 0.000000000000000000 ) ) ;
#15993=CIRCLE ( 'NONE', #19979, 2.000000000000001332 ) ;
#15997=VERTEX_POINT ( 'NONE', #4879 ) ;
#16012=DIRECTION ( 'NONE',  ( -0.4397038457472313144, 0.000000000000000000, -0.8981428216242086648 ) ) ;
#16020=ORIENTED_EDGE ( 'NONE', *, *, #11970, .F. ) ;
#16029=VECTOR ( 'NONE', #3439, 1000.000000000000227 ) ;
#16030=LINE ( 'NONE', #19094, #15458 ) ;
#16032=DIRECTION ( 'NONE',  ( -0.8981428216242028917, -0.000000000000000000, -0.4397038457472429718 ) ) ;
#16037=EDGE_CURVE ( 'NONE', #99, #12157, #2616, .T. ) ;
#16039=DIRECTION ( 'NONE',  ( 1.000000000000000000, -0.000000000000000000, -9.912705577010318154E-17 ) ) ;
#16062=DIRECTION ( 'NONE',  ( -0.000000000000000000, -1.000000000000000000, -0.000000000000000000 ) ) ;
#16065=ORIENTED_EDGE ( 'NONE', *, *, #2892, .T. ) ;
#16068=ORIENTED_EDGE ( 'NONE', *, *, #2239, .F. ) ;
#16102=DIRECTION ( 'NONE',  ( -0.000000000000000000, -1.000000000000000000, -0.000000000000000000 ) ) ;
#16132=AXIS2_PLACEMENT_3D ( 'NONE', #7584, #18383, #11374 ) ;
#16135=ORIENTED_EDGE ( 'NONE', *, *, #9891, .T. ) ;
#16139=DIRECTION ( 'NONE',  ( -1.000000000000000000, -0.000000000000000000, 1.458023040593674599E-16 ) ) ;
#16140=ORIENTED_EDGE ( 'NONE', *, *, #19495, .T. ) ;
#16141=CARTESIAN_POINT ( 'NONE',  ( 162.0000000000000000, 0.000000000000000000, -2.262479907570351121E-12 ) ) ;
#16164=AXIS2_PLACEMENT_3D ( 'NONE', #16699, #13238, #16905 ) ;
#16198=FACE_OUTER_BOUND ( 'NONE', #19017, .T. ) ;
#16216=ADVANCED_FACE ( 'NONE', ( #19785 ), #21845, .F. ) ;
#16220=CIRCLE ( 'NONE', #2618, 2.000000000000001776 ) ;
#16225=ORIENTED_EDGE ( 'NONE', *, *, #19012, .F. ) ;
#16226=CARTESIAN_POINT ( 'NONE',  ( 0.000000000000000000, 20.00000000000000000, 0.000000000000000000 ) ) ;
#16227=CIRCLE ( 'NONE', #20232, 2.000000000000001332 ) ;
#16231=CIRCLE ( 'NONE', #16962, 101.0000000000000000 ) ;
#16242=VERTEX_POINT ( 'NONE', #18551 ) ;
#16253=CARTESIAN_POINT ( 'NONE',  ( 0.000000000000000000, 29.00000000000000355, 0.000000000000000000 ) ) ;
#16255=CARTESIAN_POINT ( 'NONE',  ( 153.9999999999992610, 20.00000000000000000, -53.76161406891471017 ) ) ;
#16261=ORIENTED_EDGE ( 'NONE', *, *, #16037, .F. ) ;
#16265=VECTOR ( 'NONE', #8749, 1000.000000000000000 ) ;
#16267=VECTOR ( 'NONE', #20049, 1000.000000000000000 ) ;
#16274=VECTOR ( 'NONE', #3312, 1000.000000000000000 ) ;
#16315=LINE ( 'NONE', #21535, #443 ) ;
#16324=DIRECTION ( 'NONE',  ( 0.000000000000000000, 0.000000000000000000, -1.000000000000000000 ) ) ;
#16338=PLANE ( 'NONE',  #4464 ) ;
#16346=VERTEX_POINT ( 'NONE', #8411 ) ;
#16354=CYLINDRICAL_SURFACE ( 'NONE', #16132, 83.99999999999998579 ) ;
#16364=ORIENTED_EDGE ( 'NONE', *, *, #16556, .T. ) ;
#16400=EDGE_CURVE ( 'NONE', #10705, #20064, #5183, .T. ) ;
#16409=CARTESIAN_POINT ( 'NONE',  ( 0.000000000000000000, 45.00000000000000000, 0.000000000000000000 ) ) ;
#16412=FACE_OUTER_BOUND ( 'NONE', #12647, .T. ) ;
#16427=EDGE_CURVE ( 'NONE', #18838, #19445, #8211, .T. ) ;
#16430=LINE ( 'NONE', #12982, #3768 ) ;
#16437=DIRECTION ( 'NONE',  ( 0.000000000000000000, 1.000000000000000000, 0.000000000000000000 ) ) ;
#16444=CIRCLE ( 'NONE', #10550, 126.0000000000000000 ) ;
#16445=DIRECTION ( 'NONE',  ( -0.8981428216242028917, 0.000000000000000000, 0.4397038457472432493 ) ) ;
#16446=VERTEX_POINT ( 'NONE', #12108 ) ;
#16453=ORIENTED_EDGE ( 'NONE', *, *, #4813, .F. ) ;
#16455=CARTESIAN_POINT ( 'NONE',  ( -146.5000000000000000, 20.00000000000000000, 8.000000000000017764 ) ) ;
#16483=ORIENTED_EDGE ( 'NONE', *, *, #6427, .F. ) ;
#16484=FACE_OUTER_BOUND ( 'NONE', #5922, .T. ) ;
#16485=DIRECTION ( 'NONE',  ( -0.000000000000000000, -1.000000000000000000, -0.000000000000000000 ) ) ;
#16490=CARTESIAN_POINT ( 'NONE',  ( 0.000000000000000000, 20.00000000000000000, 0.000000000000000000 ) ) ;
#16491=DIRECTION ( 'NONE',  ( 0.4397038457472313144, 0.000000000000000000, 0.8981428216242086648 ) ) ;
#16525=EDGE_CURVE ( 'NONE', #10199, #7779, #7389, .T. ) ;
#16543=DIRECTION ( 'NONE',  ( 1.000000000000000000, 0.000000000000000000, -1.386679829960243376E-14 ) ) ;
#16548=LINE ( 'NONE', #7799, #1550 ) ;
#16550=CARTESIAN_POINT ( 'NONE',  ( -164.0000000000000000, 1.999999999999998224, -7.999999999999979572 ) ) ;
#16554=AXIS2_PLACEMENT_3D ( 'NONE', #18667, #2933, #9949 ) ;
#16556=EDGE_CURVE ( 'NONE', #15942, #16446, #2101, .T. ) ;
#16557=AXIS2_PLACEMENT_3D ( 'NONE', #19994, #5873, #19655 ) ;
#16561=EDGE_CURVE ( 'NONE', #7475, #5531, #15916, .T. ) ;
#16564=EDGE_LOOP ( 'NONE', ( #20027, #20819, #10261, #18493 ) ) ;
#16572=EDGE_CURVE ( 'NONE', #19973, #22152, #16231, .T. ) ;
#16583=TOROIDAL_SURFACE ( 'NONE', #13258, 10.00000000000000355, 2.000000000000000000 ) ;
#16588=CARTESIAN_POINT ( 'NONE',  ( -164.0000000000000000, 20.00000000000000000, 4.016841501203319170E-14 ) ) ;
#16591=CARTESIAN_POINT ( 'NONE',  ( -1.386679829960242619E-13, 18.00000000000000355, -9.999999999999994671 ) ) ;
#16592=DIRECTION ( 'NONE',  ( -0.000000000000000000, -1.000000000000000000, -0.000000000000000000 ) ) ;
#16595=VECTOR ( 'NONE', #18982, 1000.000000000000000 ) ;
#16604=ORIENTED_EDGE ( 'NONE', *, *, #19718, .T. ) ;
#16605=EDGE_CURVE ( 'NONE', #6576, #18453, #5308, .T. ) ;
#16620=DIRECTION ( 'NONE',  ( 0.8981428216242087759, 0.000000000000000000, -0.4397038457472309259 ) ) ;
#16623=CARTESIAN_POINT ( 'NONE',  ( 0.000000000000000000, 0.000000000000000000, 0.000000000000000000 ) ) ;
#16634=DIRECTION ( 'NONE',  ( 0.8981428216242030027, 0.000000000000000000, 0.4397038457472430273 ) ) ;
#16644=CARTESIAN_POINT ( 'NONE',  ( -164.0000000000000000, 20.00000000000000000, -53.76161406891256433 ) ) ;
#16667=CARTESIAN_POINT ( 'NONE',  ( 0.000000000000000000, 0.000000000000000000, 0.000000000000000000 ) ) ;
#16670=ORIENTED_EDGE ( 'NONE', *, *, #20741, .F. ) ;
#16671=CIRCLE ( 'NONE', #7848, 8.000000000000014211 ) ;
#16672=ADVANCED_FACE ( 'NONE', ( #14531 ), #22044, .T. ) ;
#16674=CARTESIAN_POINT ( 'NONE',  ( 164.0000000000000000, 1.999999999999998224, 2.250243343269062756E-12 ) ) ;
#16679=AXIS2_PLACEMENT_3D ( 'NONE', #6874, #14021, #17824 ) ;
#16684=VECTOR ( 'NONE', #21527, 1000.000000000000114 ) ;
#16694=CARTESIAN_POINT ( 'NONE',  ( -154.0000000000000000, 18.00000000000000355, 53.76161406891259986 ) ) ;
#16695=EDGE_CURVE ( 'NONE', #10082, #14514, #19834, .T. ) ;
#16696=DIRECTION ( 'NONE',  ( 0.000000000000000000, 1.000000000000000000, -0.000000000000000000 ) ) ;
#16698=ORIENTED_EDGE ( 'NONE', *, *, #6977, .F. ) ;
#16699=CARTESIAN_POINT ( 'NONE',  ( -154.0000000000000000, 18.00000000000000355, -53.76161406891256433 ) ) ;
#16700=ORIENTED_EDGE ( 'NONE', *, *, #9282, .T. ) ;
#16715=AXIS2_PLACEMENT_3D ( 'NONE', #18190, #12561, #17864 ) ;
#16719=DIRECTION ( 'NONE',  ( 0.000000000000000000, 0.000000000000000000, 1.000000000000000000 ) ) ;
#16721=DIRECTION ( 'NONE',  ( 1.000000000000000000, 0.000000000000000000, 1.362186893977296347E-14 ) ) ;
#16725=CARTESIAN_POINT ( 'NONE',  ( 54.52327687265665190, 2.000000000000000000, 111.3697098814019029 ) ) ;
#16729=AXIS2_PLACEMENT_3D ( 'NONE', #16226, #4115, #12998 ) ;
#16753=DIRECTION ( 'NONE',  ( 0.000000000000000000, 0.000000000000000000, 1.000000000000000000 ) ) ;
#16795=DIRECTION ( 'NONE',  ( -0.000000000000000000, -1.000000000000000000, -0.000000000000000000 ) ) ;
#16800=LINE ( 'NONE', #4597, #12848 ) ;
#16801=AXIS2_PLACEMENT_3D ( 'NONE', #11009, #573, #19617 ) ;
#16804=ADVANCED_FACE ( 'NONE', ( #3989, #8626 ), #16338, .T. ) ;
#16805=ORIENTED_EDGE ( 'NONE', *, *, #1098, .T. ) ;
#16817=FACE_OUTER_BOUND ( 'NONE', #9287, .T. ) ;
#16819=ORIENTED_EDGE ( 'NONE', *, *, #10688, .T. ) ;
#16863=EDGE_LOOP ( 'NONE', ( #10864, #18163 ) ) ;
#16875=ORIENTED_EDGE ( 'NONE', *, *, #10051, .T. ) ;
#16877=CYLINDRICAL_SURFACE ( 'NONE', #1114, 2.000000000000004441 ) ;
#16901=CARTESIAN_POINT ( 'NONE',  ( 0.000000000000000000, 1.999999999999998224, 124.0000000000000000 ) ) ;
#16903=DIRECTION ( 'NONE',  ( 0.000000000000000000, 0.000000000000000000, 1.000000000000000000 ) ) ;
#16905=DIRECTION ( 'NONE',  ( 0.000000000000000000, 0.000000000000000000, 1.000000000000000000 ) ) ;
#16914=PLANE ( 'NONE',  #13695 ) ;
#16917=ORIENTED_EDGE ( 'NONE', *, *, #10107, .F. ) ;
#16921=AXIS2_PLACEMENT_3D ( 'NONE', #5992, #4666, #1269 ) ;
#16925=CIRCLE ( 'NONE', #19095, 2.000000000000001332 ) ;
#16933=ORIENTED_EDGE ( 'NONE', *, *, #22105, .T. ) ;
#16935=ADVANCED_FACE ( 'NONE', ( #19516 ), #20242, .T. ) ;
#16950=FACE_OUTER_BOUND ( 'NONE', #4010, .T. ) ;
#16959=ADVANCED_FACE ( 'NONE', ( #11356 ), #20603, .T. ) ;
#16962=AXIS2_PLACEMENT_3D ( 'NONE', #6919, #13940, #7262 ) ;
#16967=EDGE_CURVE ( 'NONE', #14037, #18877, #16548, .T. ) ;
#16968=ADVANCED_FACE ( 'NONE', ( #18363 ), #19958, .T. ) ;
#16994=CIRCLE ( 'NONE', #5963, 2.000000000000000000 ) ;
#17022=FACE_OUTER_BOUND ( 'NONE', #1522, .T. ) ;
#17029=VERTEX_POINT ( 'NONE', #12151 ) ;
#17048=FACE_OUTER_BOUND ( 'NONE', #18411, .T. ) ;
#17059=LINE ( 'NONE', #8521, #13128 ) ;
#17077=CARTESIAN_POINT ( 'NONE',  ( 0.000000000000000000, 18.00000000000000355, 0.000000000000000000 ) ) ;
#17083=DIRECTION ( 'NONE',  ( -0.000000000000000000, -1.000000000000000000, -0.000000000000000000 ) ) ;
#17084=VECTOR ( 'NONE', #1622, 1000.000000000000000 ) ;
#17094=ADVANCED_FACE ( 'NONE', ( #3075 ), #10094, .T. ) ;
#17095=ORIENTED_EDGE ( 'NONE', *, *, #2951, .T. ) ;
#17105=CARTESIAN_POINT ( 'NONE',  ( 1.458023040593673859E-15, 2.000000000000000000, 9.999999999999994671 ) ) ;
#17107=ORIENTED_EDGE ( 'NONE', *, *, #16695, .T. ) ;
#17110=CARTESIAN_POINT ( 'NONE',  ( 153.9999999999992610, 0.000000000000000000, 53.76161406891468175 ) ) ;
#17121=DIRECTION ( 'NONE',  ( -0.000000000000000000, -1.000000000000000000, -0.000000000000000000 ) ) ;
#17145=LINE ( 'NONE', #8509, #18065 ) ;
#17153=ADVANCED_FACE ( 'NONE', ( #16412 ), #21640, .F. ) ;
#17154=LINE ( 'NONE', #7958, #19442 ) ;
#17160=SHAPE_REPRESENTATION_RELATIONSHIP ( 'NONE' , 'NONE' ,  #5468, #7450 ) ;
#17167=AXIS2_PLACEMENT_3D ( 'NONE', #3310, #20769, #8364 ) ;
#17173=DIRECTION ( 'NONE',  ( 0.000000000000000000, 1.000000000000000000, -0.000000000000000000 ) ) ;
#17183=DIRECTION ( 'NONE',  ( -0.000000000000000000, -1.000000000000000000, -0.000000000000000000 ) ) ;
#17189=TOROIDAL_SURFACE ( 'NONE', #12800, 124.0000000000000000, 2.000000000000000000 ) ;
#17197=ORIENTED_EDGE ( 'NONE', *, *, #7817, .F. ) ;
#17220=VERTEX_POINT ( 'NONE', #21521 ) ;
#17223=LINE ( 'NONE', #1286, #7394 ) ;
#17233=ORIENTED_EDGE ( 'NONE', *, *, #19718, .F. ) ;
#17234=DIRECTION ( 'NONE',  ( 0.000000000000000000, 0.000000000000000000, 1.000000000000000000 ) ) ;
#17244=VECTOR ( 'NONE', #3180, 1000.000000000000000 ) ;
#17253=AXIS2_PLACEMENT_3D ( 'NONE', #5925, #12963, #9737 ) ;
#17254=ORIENTED_EDGE ( 'NONE', *, *, #15886, .F. ) ;
#17262=AXIS2_PLACEMENT_3D ( 'NONE', #20942, #19337, #8748 ) ;
#17265=EDGE_CURVE ( 'NONE', #10504, #2665, #14677, .T. ) ;
#17274=( LENGTH_UNIT ( ) NAMED_UNIT ( * ) SI_UNIT ( .MILLI., .METRE. ) );
#17276=AXIS2_PLACEMENT_3D ( 'NONE', #4846, #3363, #8408 ) ;
#17288=VERTEX_POINT ( 'NONE', #8195 ) ;
#17290=CARTESIAN_POINT ( 'NONE',  ( -1.089749515181836320E-13, 20.00000000000000000, 7.999999999999994671 ) ) ;
#17309=AXIS2_PLACEMENT_3D ( 'NONE', #19438, #10600, #21266 ) ;
#17317=DIRECTION ( 'NONE',  ( 0.000000000000000000, 0.000000000000000000, 1.000000000000000000 ) ) ;
#17322=CIRCLE ( 'NONE', #20600, 78.99999999999998579 ) ;
#17340=CIRCLE ( 'NONE', #465, 78.99999999999998579 ) ;
#17343=FACE_OUTER_BOUND ( 'NONE', #1036, .T. ) ;
#17347=FACE_OUTER_BOUND ( 'NONE', #10244, .T. ) ;
#17356=ORIENTED_EDGE ( 'NONE', *, *, #7603, .F. ) ;
#17362=VECTOR ( 'NONE', #12514, 1000.000000000000000 ) ;
#17365=DIRECTION ( 'NONE',  ( -0.000000000000000000, -1.000000000000000000, -0.000000000000000000 ) ) ;
#17384=CARTESIAN_POINT ( 'NONE',  ( -90.00000000000000000, 0.000000000000000000, 8.394090934816448357E-16 ) ) ;
#17387=EDGE_CURVE ( 'NONE', #3348, #9064, #18332, .T. ) ;
#17410=ORIENTED_EDGE ( 'NONE', *, *, #6977, .T. ) ;
#17412=CYLINDRICAL_SURFACE ( 'NONE', #2670, 2.000000000000000000 ) ;
#17432=EDGE_CURVE ( 'NONE', #7572, #9599, #11364, .T. ) ;
#17438=EDGE_LOOP ( 'NONE', ( #5227, #7874, #16805, #19408 ) ) ;
#17440=ORIENTED_EDGE ( 'NONE', *, *, #22167, .F. ) ;
#17452=CARTESIAN_POINT ( 'NONE',  ( 146.5000000000000000, 18.00000000000000355, -2.025191382850354537E-12 ) ) ;
#17455=COLOUR_RGB ( '', 0.40784314, 0.44705882, 0.49803922) ;
#17458=CARTESIAN_POINT ( 'NONE',  ( 54.52327687265658085, 2.000000000000000000, -111.3697098814019171 ) ) ;
#17459=EDGE_LOOP ( 'NONE', ( #19882, #22247, #5193, #1392 ) ) ;
#17460=LINE ( 'NONE', #12168, #8026 ) ;
#17463=DIRECTION ( 'NONE',  ( 0.000000000000000000, -1.000000000000000000, 0.000000000000000000 ) ) ;
#17465=CARTESIAN_POINT ( 'NONE',  ( -146.5000000000000000, 1.999999999999998224, 2.081668171172168513E-14 ) ) ;
#17476=LINE ( 'NONE', #12310, #11423 ) ;
#17489=ORIENTED_EDGE ( 'NONE', *, *, #3252, .T. ) ;
#17491=DIRECTION ( 'NONE',  ( 0.8981428216242088869, -0.000000000000000000, -0.4397038457472309814 ) ) ;
#17516=ADVANCED_FACE ( 'NONE', ( #2928 ), #22090, .T. ) ;
#17520=EDGE_CURVE ( 'NONE', #3243, #9760, #19060, .T. ) ;
#17544=DIRECTION ( 'NONE',  ( 0.000000000000000000, 0.000000000000000000, -1.000000000000000000 ) ) ;
#17548=FACE_OUTER_BOUND ( 'NONE', #6554, .T. ) ;
#17557=CARTESIAN_POINT ( 'NONE',  ( 146.5000000000000000, 1.999999999999998224, -2.025191382850354537E-12 ) ) ;
#17558=ORIENTED_EDGE ( 'NONE', *, *, #475, .T. ) ;
#17570=EDGE_CURVE ( 'NONE', #822, #7475, #8432, .T. ) ;
#17612=EDGE_LOOP ( 'NONE', ( #6815, #1102, #19950, #2544, #20821, #13619, #19102, #7688, #19377, #16364, #18279, #21923, #13866, #10683, #14734, #4578, #982, #11060, #10129, #21566, #11491 ) ) ;
#17626=AXIS2_PLACEMENT_3D ( 'NONE', #5553, #7392, #2223 ) ;
#17634=ADVANCED_FACE ( 'NONE', ( #2573, #5895 ), #21503, .T. ) ;
#17638=ORIENTED_EDGE ( 'NONE', *, *, #20789, .T. ) ;
#17646=ORIENTED_EDGE ( 'NONE', *, *, #7815, .T. ) ;
#17648=EDGE_CURVE ( 'NONE', #6364, #3254, #10287, .T. ) ;
#17664=CIRCLE ( 'NONE', #18388, 8.000000000000014211 ) ;
#17676=EDGE_CURVE ( 'NONE', #7464, #11795, #516, .T. ) ;
#17703=CARTESIAN_POINT ( 'NONE',  ( 1.236893267138826732E-14, 37.00000000000000711, 101.0000000000000000 ) ) ;
#17709=DIRECTION ( 'NONE',  ( 0.8981428216242086648, 1.300010802462040013E-16, -0.4397038457472312589 ) ) ;
#17732=AXIS2_PLACEMENT_3D ( 'NONE', #16253, #2674, #2327 ) ;
#17735=FACE_OUTER_BOUND ( 'NONE', #8530, .T. ) ;
#17738=CARTESIAN_POINT ( 'NONE',  ( 153.9999999999992610, 1.999999999999998224, 53.76161406891468175 ) ) ;
#17744=EDGE_CURVE ( 'NONE', #7438, #1225, #17154, .T. ) ;
#17754=ORIENTED_EDGE ( 'NONE', *, *, #19715, .F. ) ;
#17755=CIRCLE ( 'NONE', #3423, 2.000000000000001332 ) ;
#17765=CYLINDRICAL_SURFACE ( 'NONE', #4158, 8.000000000000003553 ) ;
#17768=DIRECTION ( 'NONE',  ( 0.000000000000000000, 0.000000000000000000, 1.000000000000000000 ) ) ;
#17784=VECTOR ( 'NONE', #1025, 1000.000000000000000 ) ;
#17788=CARTESIAN_POINT ( 'NONE',  ( 161.9999999999998579, 0.000000000000000000, -10.00000000000224176 ) ) ;
#17806=AXIS2_PLACEMENT_3D ( 'NONE', #21387, #3832, #12456 ) ;
#17824=DIRECTION ( 'NONE',  ( -1.387778780781445044E-14, 0.000000000000000000, 1.000000000000000000 ) ) ;
#17831=DIRECTION ( 'NONE',  ( -0.000000000000000000, -1.000000000000000000, -0.000000000000000000 ) ) ;
#17842=SHAPE_DEFINITION_REPRESENTATION ( #11206, #5468 ) ;
#17848=DIRECTION ( 'NONE',  ( -1.372099599554306628E-14, 0.000000000000000000, 1.000000000000000000 ) ) ;
#17862=EDGE_LOOP ( 'NONE', ( #8890, #5487, #4327, #4478 ) ) ;
#17864=DIRECTION ( 'NONE',  ( 0.4397038457472424167, 0.000000000000000000, -0.8981428216242032248 ) ) ;
#17895=FACE_OUTER_BOUND ( 'NONE', #6761, .T. ) ;
#17907=FACE_OUTER_BOUND ( 'NONE', #8747, .T. ) ;
#17909=DIRECTION ( 'NONE',  ( 1.387778780781444571E-14, 0.000000000000000000, -1.000000000000000000 ) ) ;
#17917=EDGE_LOOP ( 'NONE', ( #20546, #14738, #21859, #5455 ) ) ;
#17931=CARTESIAN_POINT ( 'NONE',  ( 0.000000000000000000, 45.00000000000000000, 0.000000000000000000 ) ) ;
#17932=CARTESIAN_POINT ( 'NONE',  ( 153.9999999999992610, 20.00000000000000000, -53.76161406891471017 ) ) ;
#17938=EDGE_CURVE ( 'NONE', #168, #8602, #16800, .T. ) ;
#17945=EDGE_CURVE ( 'NONE', #7906, #10199, #13693, .T. ) ;
#17966=DIRECTION ( 'NONE',  ( 2.449293598294706414E-16, 0.000000000000000000, 1.000000000000000000 ) ) ;
#17969=VERTEX_POINT ( 'NONE', #10009 ) ;
#17991=EDGE_CURVE ( 'NONE', #2134, #1879, #10355, .T. ) ;
#18026=ORIENTED_EDGE ( 'NONE', *, *, #632, .T. ) ;
#18032=AXIS2_PLACEMENT_3D ( 'NONE', #8210, #20368, #9925 ) ;
#18044=FACE_OUTER_BOUND ( 'NONE', #3734, .T. ) ;
#18047=ORIENTED_EDGE ( 'NONE', *, *, #11609, .F. ) ;
#18062=FACE_OUTER_BOUND ( 'NONE', #22587, .T. ) ;
#18065=VECTOR ( 'NONE', #6791, 1000.000000000000000 ) ;
#18069=ORIENTED_EDGE ( 'NONE', *, *, #19692, .F. ) ;
#18082=CARTESIAN_POINT ( 'NONE',  ( -162.0000000000000000, 20.00000000000000000, 3.967855629237424480E-14 ) ) ;
#18088=VECTOR ( 'NONE', #4584, 1000.000000000000000 ) ;
#18108=CARTESIAN_POINT ( 'NONE',  ( 146.4999999999998579, 2.000000000000000000, -10.00000000000202682 ) ) ;
#18111=AXIS2_PLACEMENT_3D ( 'NONE', #8282, #11625, #13471 ) ;
#18123=VECTOR ( 'NONE', #6391, 1000.000000000000000 ) ;
#18127=DIRECTION ( 'NONE',  ( -0.000000000000000000, -1.000000000000000000, 0.000000000000000000 ) ) ;
#18138=CIRCLE ( 'NONE', #21044, 83.99999999999998579 ) ;
#18146=ORIENTED_EDGE ( 'NONE', *, *, #818, .F. ) ;
#18156=AXIS2_PLACEMENT_3D ( 'NONE', #2919, #9931, #22200 ) ;
#18158=DIRECTION ( 'NONE',  ( 0.4397038457472493556, 0.000000000000000000, -0.8981428216241997831 ) ) ;
#18163=ORIENTED_EDGE ( 'NONE', *, *, #13445, .T. ) ;
#18177=VECTOR ( 'NONE', #8709, 1000.000000000000000 ) ;
#18178=CARTESIAN_POINT ( 'NONE',  ( 0.000000000000000000, 0.000000000000000000, 0.000000000000000000 ) ) ;
#18190=CARTESIAN_POINT ( 'NONE',  ( -54.52327687265812273, 18.00000000000000355, 111.3697098814011923 ) ) ;
#18191=DIRECTION ( 'NONE',  ( -0.000000000000000000, -1.000000000000000000, -0.000000000000000000 ) ) ;
#18211=AXIS2_PLACEMENT_3D ( 'NONE', #15193, #16696, #20206 ) ;
#18242=ORIENTED_EDGE ( 'NONE', *, *, #17265, .T. ) ;
#18246=CYLINDRICAL_SURFACE ( 'NONE', #10357, 78.99999999999998579 ) ;
#18248=CIRCLE ( 'NONE', #11280, 126.0000000000000000 ) ;
#18257=DIRECTION ( 'NONE',  ( 0.000000000000000000, 1.000000000000000000, -0.000000000000000000 ) ) ;
#18259=FACE_OUTER_BOUND ( 'NONE', #21918, .T. ) ;
#18267=EDGE_CURVE ( 'NONE', #21547, #14045, #7678, .T. ) ;
#18269=DIRECTION ( 'NONE',  ( -0.4397038457472424167, 0.000000000000000000, -0.8981428216242032248 ) ) ;
#18271=PRODUCT_CONTEXT ( 'NONE', #5421, 'mechanical' ) ;
#18272=VECTOR ( 'NONE', #4370, 1000.000000000000000 ) ;
#18274=CARTESIAN_POINT ( 'NONE',  ( 54.52327687265662348, 18.00000000000000355, -111.3697098814019313 ) ) ;
#18278=CARTESIAN_POINT ( 'NONE',  ( -162.0000000000000000, 20.00000000000000000, -53.76161406891256433 ) ) ;
#18279=ORIENTED_EDGE ( 'NONE', *, *, #13327, .T. ) ;
#18293=ORIENTED_EDGE ( 'NONE', *, *, #22387, .F. ) ;
#18297=ORIENTED_EDGE ( 'NONE', *, *, #7942, .F. ) ;
#18304=ORIENTED_EDGE ( 'NONE', *, *, #3141, .F. ) ;
#18320=DIRECTION ( 'NONE',  ( 0.000000000000000000, 0.000000000000000000, -1.000000000000000000 ) ) ;
#18332=CIRCLE ( 'NONE', #6591, 83.99999999999998579 ) ;
#18334=CYLINDRICAL_SURFACE ( 'NONE', #17253, 2.000000000000001332 ) ;
#18346=PRODUCT ( 'Lower Angular Base Cradle Segment', 'Lower Angular Base Cradle Segment', '', ( #18271 ) ) ;
#18348=LINE ( 'NONE', #9750, #8493 ) ;
#18363=FACE_OUTER_BOUND ( 'NONE', #1829, .T. ) ;
#18367=DIRECTION ( 'NONE',  ( -1.372099599554306628E-14, 0.000000000000000000, 1.000000000000000000 ) ) ;
#18382=ORIENTED_EDGE ( 'NONE', *, *, #11458, .F. ) ;
#18383=DIRECTION ( 'NONE',  ( -0.000000000000000000, -1.000000000000000000, -0.000000000000000000 ) ) ;
#18388=AXIS2_PLACEMENT_3D ( 'NONE', #8278, #8376, #17234 ) ;
#18392=DIRECTION ( 'NONE',  ( -0.000000000000000000, -1.000000000000000000, -0.000000000000000000 ) ) ;
#18410=EDGE_CURVE ( 'NONE', #10488, #1018, #17322, .T. ) ;
#18411=EDGE_LOOP ( 'NONE', ( #8518, #4002, #13330, #16068 ) ) ;
#18438=CIRCLE ( 'NONE', #15147, 126.0000000000000000 ) ;
#18453=VERTEX_POINT ( 'NONE', #7537 ) ;
#18462=DIRECTION ( 'NONE',  ( -0.000000000000000000, -1.000000000000000000, 0.000000000000000000 ) ) ;
#18490=CARTESIAN_POINT ( 'NONE',  ( 0.000000000000000000, 23.00000000000000000, -120.0000000000000000 ) ) ;
#18493=ORIENTED_EDGE ( 'NONE', *, *, #20741, .T. ) ;
#18505=DIRECTION ( 'NONE',  ( 0.000000000000000000, 1.000000000000000000, -0.000000000000000000 ) ) ;
#18506=LINE ( 'NONE', #2767, #18088 ) ;
#18516=CARTESIAN_POINT ( 'NONE',  ( 153.9999999999992610, 18.00000000000000355, 53.76161406891468175 ) ) ;
#18518=CYLINDRICAL_SURFACE ( 'NONE', #8687, 10.99999999999999289 ) ;
#18521=CARTESIAN_POINT ( 'NONE',  ( 0.000000000000000000, 0.000000000000000000, 0.000000000000000000 ) ) ;
#18551=CARTESIAN_POINT ( 'NONE',  ( 0.000000000000000000, 45.00000000000000711, -96.00000000000000000 ) ) ;
#18579=VERTEX_POINT ( 'NONE', #12002 ) ;
#18582=DIRECTION ( 'NONE',  ( 1.386679829960243376E-14, -0.000000000000000000, 1.000000000000000000 ) ) ;
#18597=LINE ( 'NONE', #20317, #1079 ) ;
#18613=CARTESIAN_POINT ( 'NONE',  ( 54.52327687265664480, 0.000000000000000000, 111.3697098814019029 ) ) ;
#18617=EDGE_LOOP ( 'NONE', ( #16140, #16698, #10671, #13083 ) ) ;
#18620=EDGE_LOOP ( 'NONE', ( #3129, #17254, #184, #20957, #3267 ) ) ;
#18624=EDGE_CURVE ( 'NONE', #18579, #7423, #18438, .T. ) ;
#18630=EDGE_CURVE ( 'NONE', #14680, #1627, #19739, .T. ) ;
#18646=ORIENTED_EDGE ( 'NONE', *, *, #9642, .T. ) ;
#18654=CARTESIAN_POINT ( 'NONE',  ( 163.9999999999992610, 20.00000000000000000, -53.76161406891485228 ) ) ;
#18661=DIRECTION ( 'NONE',  ( 1.000000000000000000, -0.000000000000000000, 1.362186893977296347E-14 ) ) ;
#18667=CARTESIAN_POINT ( 'NONE',  ( -90.00000000000000000, 45.00100000000000477, 8.394090934816448357E-16 ) ) ;
#18680=CIRCLE ( 'NONE', #6937, 2.000000000000000000 ) ;
#18687=ADVANCED_FACE ( 'NONE', ( #18062 ), #17412, .T. ) ;
#18702=DIRECTION ( 'NONE',  ( 0.000000000000000000, 0.000000000000000000, 1.000000000000000000 ) ) ;
#18710=CARTESIAN_POINT ( 'NONE',  ( -54.52327687265815115, 20.00000000000000000, -111.3697098814011781 ) ) ;
#18719=ORIENTED_EDGE ( 'NONE', *, *, #12375, .T. ) ;
#18722=LINE ( 'NONE', #13360, #10053 ) ;
#18727=FACE_OUTER_BOUND ( 'NONE', #10280, .T. ) ;
#18737=EDGE_CURVE ( 'NONE', #724, #8008, #17340, .T. ) ;
#18747=DIRECTION ( 'NONE',  ( 1.362186893977296031E-14, 0.000000000000000000, -1.000000000000000000 ) ) ;
#18769=ORIENTED_EDGE ( 'NONE', *, *, #7942, .T. ) ;
#18784=DIRECTION ( 'NONE',  ( 0.000000000000000000, 1.000000000000000000, -0.000000000000000000 ) ) ;
#18805=CIRCLE ( 'NONE', #17732, 101.0000000000000000 ) ;
#18809=ADVANCED_FACE ( 'NONE', ( #17347 ), #13891, .T. ) ;
#18812=AXIS2_PLACEMENT_3D ( 'NONE', #21660, #18582, #16543 ) ;
#18815=ORIENTED_EDGE ( 'NONE', *, *, #19238, .F. ) ;
#18821=DIRECTION ( 'NONE',  ( 0.000000000000000000, 0.000000000000000000, -1.000000000000000000 ) ) ;
#18828=AXIS2_PLACEMENT_3D ( 'NONE', #15694, #10857, #7277 ) ;
#18838=VERTEX_POINT ( 'NONE', #22577 ) ;
#18860=AXIS2_PLACEMENT_3D ( 'NONE', #5266, #17709, #14148 ) ;
#18875=ORIENTED_EDGE ( 'NONE', *, *, #11055, .T. ) ;
#18877=VERTEX_POINT ( 'NONE', #8471 ) ;
#18883=CARTESIAN_POINT ( 'NONE',  ( -1.390668784055079922E-14, 45.00000000000000000, -110.1134477342067299 ) ) ;
#18911=PRODUCT_DEFINITION_CONTEXT ( 'detailed design', #21130, 'design' ) ;
#18918=FACE_OUTER_BOUND ( 'NONE', #7263, .T. ) ;
#18920=EDGE_CURVE ( 'NONE', #19445, #7377, #4116, .T. ) ;
#18931=EDGE_LOOP ( 'NONE', ( #16933, #5190, #7037, #16020 ) ) ;
#18934=LINE ( 'NONE', #3191, #6702 ) ;
#18935=DIRECTION ( 'NONE',  ( -0.8981428216242088869, 0.000000000000000000, -0.4397038457472307593 ) ) ;
#18939=LINE ( 'NONE', #22360, #20679 ) ;
#18947=ORIENTED_EDGE ( 'NONE', *, *, #16695, .F. ) ;
#18951=EDGE_CURVE ( 'NONE', #9416, #3659, #21220, .T. ) ;
#18982=DIRECTION ( 'NONE',  ( 2.449293598294706414E-16, -0.000000000000000000, 1.000000000000000000 ) ) ;
#18989=ORIENTED_EDGE ( 'NONE', *, *, #2832, .F. ) ;
#18992=AXIS2_PLACEMENT_3D ( 'NONE', #1687, #20505, #8331 ) ;
#18996=CARTESIAN_POINT ( 'NONE',  ( 161.9999999999998579, 20.00000000000000000, -10.00000000000224176 ) ) ;
#19002=EDGE_CURVE ( 'NONE', #19051, #12157, #8187, .T. ) ;
#19008=ORIENTED_EDGE ( 'NONE', *, *, #15975, .F. ) ;
#19012=EDGE_CURVE ( 'NONE', #5068, #1879, #4102, .T. ) ;
#19014=LINE ( 'NONE', #3276, #12448 ) ;
#19017=EDGE_LOOP ( 'NONE', ( #12788, #13299 ) ) ;
#19020=CARTESIAN_POINT ( 'NONE',  ( -154.0000000000000000, 1.999999999999998224, 53.76161406891259986 ) ) ;
#19026=ORIENTED_EDGE ( 'NONE', *, *, #14135, .T. ) ;
#19039=VECTOR ( 'NONE', #468, 1000.000000000000000 ) ;
#19048=VERTEX_POINT ( 'NONE', #21335 ) ;
#19051=VERTEX_POINT ( 'NONE', #2282 ) ;
#19057=AXIS2_PLACEMENT_3D ( 'NONE', #5827, #21125, #18158 ) ;
#19060=CIRCLE ( 'NONE', #12832, 2.000000000000001776 ) ;
#19070=LINE ( 'NONE', #10364, #11900 ) ;
#19087=CARTESIAN_POINT ( 'NONE',  ( 9.674709713264089326E-15, 0.000000000000000000, 78.99999999999998579 ) ) ;
#19094=CARTESIAN_POINT ( 'NONE',  ( 1.166418432474939088E-15, 1.999999999999998224, 7.999999999999994671 ) ) ;
#19095=AXIS2_PLACEMENT_3D ( 'NONE', #19162, #5604, #7002 ) ;
#19102=ORIENTED_EDGE ( 'NONE', *, *, #1431, .T. ) ;
#19122=VERTEX_POINT ( 'NONE', #21996 ) ;
#19143=EDGE_LOOP ( 'NONE', ( #4064, #19249, #15753, #18382 ) ) ;
#19147=CARTESIAN_POINT ( 'NONE',  ( 161.9999999999998579, 20.00000000000000000, 10.00000000000220091 ) ) ;
#19159=EDGE_CURVE ( 'NONE', #7061, #5236, #10010, .T. ) ;
#19161=CARTESIAN_POINT ( 'NONE',  ( -158.3970384574724335, 18.00000000000000355, -62.74304228515459414 ) ) ;
#19162=CARTESIAN_POINT ( 'NONE',  ( 157.5176307659771169, 2.000000000000000000, 60.94675664190834397 ) ) ;
#19176=TOROIDAL_SURFACE ( 'NONE', #9276, 118.0000000000000000, 2.000000000000000000 ) ;
#19179=CARTESIAN_POINT ( 'NONE',  ( -158.3970384574724051, 20.00000000000000000, 62.74304228515463677 ) ) ;
#19180=EDGE_CURVE ( 'NONE', #10707, #6260, #16430, .T. ) ;
#19193=AXIS2_PLACEMENT_3D ( 'NONE', #22282, #16721, #18747 ) ;
#19203=LINE ( 'NONE', #19087, #10424 ) ;
#19215=ORIENTED_EDGE ( 'NONE', *, *, #17520, .T. ) ;
#19224=VECTOR ( 'NONE', #83, 1000.000000000000000 ) ;
#19238=EDGE_CURVE ( 'NONE', #6364, #10233, #11487, .T. ) ;
#19244=ORIENTED_EDGE ( 'NONE', *, *, #4636, .T. ) ;
#19249=ORIENTED_EDGE ( 'NONE', *, *, #19012, .T. ) ;
#19256=VERTEX_POINT ( 'NONE', #2624 ) ;
#19262=ORIENTED_EDGE ( 'NONE', *, *, #14703, .F. ) ;
#19280=CIRCLE ( 'NONE', #7174, 8.000000000000014211 ) ;
#19297=LINE ( 'NONE', #11944, #17784 ) ;
#19298=EDGE_CURVE ( 'NONE', #8602, #2955, #479, .T. ) ;
#19312=DIRECTION ( 'NONE',  ( 0.000000000000000000, 0.000000000000000000, -1.000000000000000000 ) ) ;
#19313=ORIENTED_EDGE ( 'NONE', *, *, #21029, .T. ) ;
#19326=EDGE_CURVE ( 'NONE', #14680, #20163, #16994, .T. ) ;
#19337=DIRECTION ( 'NONE',  ( -1.000000000000000000, 0.000000000000000000, -1.372099599554306628E-14 ) ) ;
#19338=DIRECTION ( 'NONE',  ( -0.000000000000000000, -1.000000000000000000, -0.000000000000000000 ) ) ;
#19341=CARTESIAN_POINT ( 'NONE',  ( -55.40268456415265774, 20.00000000000000000, -113.1659955246495741 ) ) ;
#19350=EDGE_CURVE ( 'NONE', #18453, #21547, #6622, .T. ) ;
#19377=ORIENTED_EDGE ( 'NONE', *, *, #10333, .T. ) ;
#19385=ORIENTED_EDGE ( 'NONE', *, *, #19495, .F. ) ;
#19393=ORIENTED_EDGE ( 'NONE', *, *, #22105, .F. ) ;
#19408=ORIENTED_EDGE ( 'NONE', *, *, #6195, .F. ) ;
#19411=ORIENTED_EDGE ( 'NONE', *, *, #19298, .T. ) ;
#19423=DIRECTION ( 'NONE',  ( 0.000000000000000000, 0.000000000000000000, 1.000000000000000000 ) ) ;
#19433=LINE ( 'NONE', #14065, #22079 ) ;
#19438=CARTESIAN_POINT ( 'NONE',  ( -154.0000000000000000, 20.00000000000000000, -53.76161406891256433 ) ) ;
#19442=VECTOR ( 'NONE', #6478, 1000.000000000000000 ) ;
#19445=VERTEX_POINT ( 'NONE', #14460 ) ;
#19471=AXIS2_PLACEMENT_3D ( 'NONE', #21484, #4482, #11169 ) ;
#19475=CIRCLE ( 'NONE', #20939, 126.0000000000000000 ) ;
#19495=EDGE_CURVE ( 'NONE', #8011, #8602, #17755, .T. ) ;
#19497=ORIENTED_EDGE ( 'NONE', *, *, #11629, .F. ) ;
#19503=DIRECTION ( 'NONE',  ( -0.000000000000000000, -1.000000000000000000, -0.000000000000000000 ) ) ;
#19516=FACE_OUTER_BOUND ( 'NONE', #4935, .T. ) ;
#19517=CYLINDRICAL_SURFACE ( 'NONE', #20693, 2.000000000000001776 ) ;
#19534=CIRCLE ( 'NONE', #17167, 2.000000000000004441 ) ;
#19570=AXIS2_PLACEMENT_3D ( 'NONE', #9545, #20090, #11271 ) ;
#19590=ORIENTED_EDGE ( 'NONE', *, *, #2650, .F. ) ;
#19597=AXIS2_PLACEMENT_3D ( 'NONE', #16409, #11331, #654 ) ;
#19617=DIRECTION ( 'NONE',  ( 0.000000000000000000, 0.000000000000000000, -1.000000000000000000 ) ) ;
#19621=ORIENTED_EDGE ( 'NONE', *, *, #20150, .F. ) ;
#19623=DIRECTION ( 'NONE',  ( 0.000000000000000000, 1.000000000000000000, 0.000000000000000000 ) ) ;
#19629=FACE_OUTER_BOUND ( 'NONE', #18617, .T. ) ;
#19635=CIRCLE ( 'NONE', #15284, 124.0000000000000000 ) ;
#19637=ORIENTED_EDGE ( 'NONE', *, *, #10688, .F. ) ;
#19644=ADVANCED_FACE ( 'NONE', ( #3042 ), #20827, .T. ) ;
#19655=DIRECTION ( 'NONE',  ( 0.000000000000000000, 0.000000000000000000, 1.000000000000000000 ) ) ;
#19673=DIRECTION ( 'NONE',  ( 0.000000000000000000, -1.000000000000000000, 0.000000000000000000 ) ) ;
#19681=ORIENTED_EDGE ( 'NONE', *, *, #669, .F. ) ;
#19692=EDGE_CURVE ( 'NONE', #1018, #724, #15137, .T. ) ;
#19699=DIRECTION ( 'NONE',  ( 0.8981428216242032248, 0.000000000000000000, 0.4397038457472424167 ) ) ;
#19711=DIRECTION ( 'NONE',  ( -0.000000000000000000, -1.000000000000000000, 0.000000000000000000 ) ) ;
#19713=ORIENTED_EDGE ( 'NONE', *, *, #16556, .F. ) ;
#19714=AXIS2_PLACEMENT_3D ( 'NONE', #957, #4602, #4700 ) ;
#19715=EDGE_CURVE ( 'NONE', #168, #10199, #7463, .T. ) ;
#19718=EDGE_CURVE ( 'NONE', #2916, #3937, #12978, .T. ) ;
#19722=CARTESIAN_POINT ( 'NONE',  ( 0.000000000000000000, 45.00000000000000000, 0.000000000000000000 ) ) ;
#19730=ORIENTED_EDGE ( 'NONE', *, *, #11683, .T. ) ;
#19732=CIRCLE ( 'NONE', #9851, 10.99999999999999289 ) ;
#19739=LINE ( 'NONE', #16455, #16265 ) ;
#19740=ORIENTED_EDGE ( 'NONE', *, *, #4813, .T. ) ;
#19741=CARTESIAN_POINT ( 'NONE',  ( -154.0000000000000000, 1.999999999999998224, 53.76161406891259986 ) ) ;
#19745=DIRECTION ( 'NONE',  ( 0.000000000000000000, 0.000000000000000000, -1.000000000000000000 ) ) ;
#19748=EDGE_CURVE ( 'NONE', #11124, #21547, #10398, .T. ) ;
#19755=AXIS2_PLACEMENT_3D ( 'NONE', #2307, #9308, #15064 ) ;
#19780=DIRECTION ( 'NONE',  ( 1.000000000000000000, 0.000000000000000000, -0.000000000000000000 ) ) ;
#19785=FACE_OUTER_BOUND ( 'NONE', #17917, .T. ) ;
#19793=ADVANCED_FACE ( 'NONE', ( #20945 ), #21397, .T. ) ;
#19814=CARTESIAN_POINT ( 'NONE',  ( -162.0000000000000000, 0.000000000000000000, 10.00000000000001776 ) ) ;
#19828=ORIENTED_EDGE ( 'NONE', *, *, #18410, .F. ) ;
#19834=CIRCLE ( 'NONE', #9962, 10.99999999999999289 ) ;
#19847=CARTESIAN_POINT ( 'NONE',  ( -163.1715728752537871, -3.619427204118298386E-16, 8.828427124746209387 ) ) ;
#19857=CYLINDRICAL_SURFACE ( 'NONE', #20112, 2.000000000000004441 ) ;
#19858=CARTESIAN_POINT ( 'NONE',  ( 0.000000000000000000, 29.00000000000000711, 0.000000000000000000 ) ) ;
#19859=VERTEX_POINT ( 'NONE', #3496 ) ;
#19865=EDGE_CURVE ( 'NONE', #9211, #3408, #8649, .T. ) ;
#19867=DIRECTION ( 'NONE',  ( 0.000000000000000000, 1.000000000000000000, -0.000000000000000000 ) ) ;
#19872=FACE_OUTER_BOUND ( 'NONE', #18620, .T. ) ;
#19876=PLANE ( 'NONE',  #13622 ) ;
#19878=ORIENTED_EDGE ( 'NONE', *, *, #9642, .F. ) ;
#19882=ORIENTED_EDGE ( 'NONE', *, *, #16037, .T. ) ;
#19883=CARTESIAN_POINT ( 'NONE',  ( -162.0000000000000000, 20.00000000000000000, 0.000000000000000000 ) ) ;
#19893=EDGE_LOOP ( 'NONE', ( #9255, #14647, #21553, #15018 ) ) ;
#19911=CARTESIAN_POINT ( 'NONE',  ( 157.5176307659770885, 2.000000000000000000, -60.94675664190840081 ) ) ;
#19916=ADVANCED_FACE ( 'NONE', ( #7515 ), #22474, .T. ) ;
#19919=CIRCLE ( 'NONE', #11884, 78.99999999999998579 ) ;
#19941=ORIENTED_EDGE ( 'NONE', *, *, #4092, .F. ) ;
#19950=ORIENTED_EDGE ( 'NONE', *, *, #10461, .T. ) ;
#19951=CIRCLE ( 'NONE', #19597, 110.1134477342067157 ) ;
#19958=PLANE ( 'NONE',  #8153 ) ;
#19973=VERTEX_POINT ( 'NONE', #4168 ) ;
#19979=AXIS2_PLACEMENT_3D ( 'NONE', #6885, #22374, #3451 ) ;
#19985=FACE_OUTER_BOUND ( 'NONE', #6711, .T. ) ;
#19994=CARTESIAN_POINT ( 'NONE',  ( 0.000000000000000000, 25.00000000000000000, 0.000000000000000000 ) ) ;
#20011=DIRECTION ( 'NONE',  ( 0.000000000000000000, 1.000000000000000000, 0.000000000000000000 ) ) ;
#20027=ORIENTED_EDGE ( 'NONE', *, *, #15175, .T. ) ;
#20029=ORIENTED_EDGE ( 'NONE', *, *, #11629, .T. ) ;
#20049=DIRECTION ( 'NONE',  ( -0.000000000000000000, -1.000000000000000000, -0.000000000000000000 ) ) ;
#20064=VERTEX_POINT ( 'NONE', #6363 ) ;
#20078=DIRECTION ( 'NONE',  ( -1.000000000000000000, 0.000000000000000000, 1.386679829960243376E-14 ) ) ;
#20090=DIRECTION ( 'NONE',  ( 0.000000000000000000, 1.000000000000000000, -0.000000000000000000 ) ) ;
#20112=AXIS2_PLACEMENT_3D ( 'NONE', #18274, #5849, #9662 ) ;
#20121=ADVANCED_FACE ( 'NONE', ( #17735 ), #8727, .T. ) ;
#20131=DIRECTION ( 'NONE',  ( -2.449293598294706414E-16, -0.000000000000000000, -1.000000000000000000 ) ) ;
#20138=FACE_OUTER_BOUND ( 'NONE', #15007, .T. ) ;
#20142=CARTESIAN_POINT ( 'NONE',  ( -157.5176307659779411, 2.000000000000000000, -60.94675664190620523 ) ) ;
#20147=LINE ( 'NONE', #16644, #912 ) ;
#20150=EDGE_CURVE ( 'NONE', #2955, #3529, #254, .T. ) ;
#20156=EDGE_LOOP ( 'NONE', ( #728, #4790, #3492, #13129 ) ) ;
#20163=VERTEX_POINT ( 'NONE', #21038 ) ;
#20170=EDGE_CURVE ( 'NONE', #1018, #10488, #19919, .T. ) ;
#20171=CARTESIAN_POINT ( 'NONE',  ( 0.000000000000000000, 0.000000000000000000, 0.000000000000000000 ) ) ;
#20172=AXIS2_PLACEMENT_3D ( 'NONE', #22215, #1566, #22540 ) ;
#20204=LINE ( 'NONE', #4471, #1573 ) ;
#20206=DIRECTION ( 'NONE',  ( 0.000000000000000000, 0.000000000000000000, 1.000000000000000000 ) ) ;
#20209=ORIENTED_EDGE ( 'NONE', *, *, #1085, .F. ) ;
#20214=DIRECTION ( 'NONE',  ( -2.775557561562888984E-15, 0.000000000000000000, 1.000000000000000000 ) ) ;
#20220=DIRECTION ( 'NONE',  ( 0.000000000000000000, 0.000000000000000000, 1.000000000000000000 ) ) ;
#20232=AXIS2_PLACEMENT_3D ( 'NONE', #15967, #19699, #3967 ) ;
#20242=TOROIDAL_SURFACE ( 'NONE', #1909, 10.00000000000000355, 2.000000000000000000 ) ;
#20258=CARTESIAN_POINT ( 'NONE',  ( 0.000000000000000000, 45.00000000000000711, 0.000000000000000000 ) ) ;
#20272=CARTESIAN_POINT ( 'NONE',  ( 163.9999999999998863, 18.00000000000000355, -8.000000000002268408 ) ) ;
#20276=FACE_OUTER_BOUND ( 'NONE', #20370, .T. ) ;
#20279=EDGE_CURVE ( 'NONE', #2837, #10707, #1971, .T. ) ;
#20306=ORIENTED_EDGE ( 'NONE', *, *, #14210, .F. ) ;
#20308=CARTESIAN_POINT ( 'NONE',  ( -154.0000000000000000, 18.00000000000000355, -53.76161406891256433 ) ) ;
#20313=LINE ( 'NONE', #4791, #17244 ) ;
#20317=CARTESIAN_POINT ( 'NONE',  ( 161.9999999999992610, 20.00000000000000000, -53.76161406891482386 ) ) ;
#20321=VECTOR ( 'NONE', #8642, 1000.000000000000000 ) ;
#20346=CARTESIAN_POINT ( 'NONE',  ( -162.0000000000000000, 2.000000000000000000, -53.76161406891256433 ) ) ;
#20348=ORIENTED_EDGE ( 'NONE', *, *, #11607, .T. ) ;
#20355=DIRECTION ( 'NONE',  ( -1.362186893977296031E-14, 0.000000000000000000, 1.000000000000000000 ) ) ;
#20368=DIRECTION ( 'NONE',  ( 1.396592535537253658E-14, 0.000000000000000000, 1.000000000000000000 ) ) ;
#20370=EDGE_LOOP ( 'NONE', ( #20348, #19713, #10579, #20209 ) ) ;
#20385=FACE_OUTER_BOUND ( 'NONE', #14352, .T. ) ;
#20388=ORIENTED_EDGE ( 'NONE', *, *, #11529, .T. ) ;
#20393=EDGE_LOOP ( 'NONE', ( #10469, #9381, #2694, #4880 ) ) ;
#20396=DIRECTION ( 'NONE',  ( 0.000000000000000000, 0.000000000000000000, 1.000000000000000000 ) ) ;
#20400=DIRECTION ( 'NONE',  ( -0.4397038457472307593, 0.000000000000000000, 0.8981428216242088869 ) ) ;
#20421=EDGE_LOOP ( 'NONE', ( #14, #4964, #20532, #6865 ) ) ;
#20440=VECTOR ( 'NONE', #17831, 1000.000000000000000 ) ;
#20452=ORIENTED_EDGE ( 'NONE', *, *, #11745, .T. ) ;
#20472=VECTOR ( 'NONE', #13173, 1000.000000000000000 ) ;
#20501=ADVANCED_FACE ( 'NONE', ( #11719 ), #13390, .T. ) ;
#20505=DIRECTION ( 'NONE',  ( -0.000000000000000000, -1.000000000000000000, -0.000000000000000000 ) ) ;
#20513=DIRECTION ( 'NONE',  ( 0.000000000000000000, 1.000000000000000000, -0.000000000000000000 ) ) ;
#20519=DIRECTION ( 'NONE',  ( -0.000000000000000000, -1.000000000000000000, -0.000000000000000000 ) ) ;
#20526=VECTOR ( 'NONE', #5769, 1000.000000000000000 ) ;
#20532=ORIENTED_EDGE ( 'NONE', *, *, #7445, .F. ) ;
#20540=CARTESIAN_POINT ( 'NONE',  ( 9.674709713264089326E-15, 37.00000000000000711, 78.99999999999998579 ) ) ;
#20546=ORIENTED_EDGE ( 'NONE', *, *, #3149, .F. ) ;
#20561=CIRCLE ( 'NONE', #7744, 10.00000000000001599 ) ;
#20562=ORIENTED_EDGE ( 'NONE', *, *, #21304, .T. ) ;
#20571=CARTESIAN_POINT ( 'NONE',  ( -162.0000000000000000, 0.000000000000000000, 53.76161406891260697 ) ) ;
#20598=EDGE_LOOP ( 'NONE', ( #3994, #19411, #14293, #13376 ) ) ;
#20600=AXIS2_PLACEMENT_3D ( 'NONE', #7760, #13174, #18320 ) ;
#20601=ORIENTED_EDGE ( 'NONE', *, *, #561, .T. ) ;
#20603=TOROIDAL_SURFACE ( 'NONE', #2995, 124.0000000000000000, 2.000000000000000000 ) ;
#20604=FACE_OUTER_BOUND ( 'NONE', #5076, .T. ) ;
#20609=EDGE_CURVE ( 'NONE', #10751, #9038, #10983, .T. ) ;
#20620=AXIS2_PLACEMENT_3D ( 'NONE', #13555, #10109, #1714 ) ;
#20623=EDGE_CURVE ( 'NONE', #5930, #7993, #7082, .T. ) ;
#20626=DIRECTION ( 'NONE',  ( -0.000000000000000000, -1.000000000000000000, -0.000000000000000000 ) ) ;
#20632=AXIS2_PLACEMENT_3D ( 'NONE', #7564, #19711, #3652 ) ;
#20679=VECTOR ( 'NONE', #8273, 1000.000000000000000 ) ;
#20693=AXIS2_PLACEMENT_3D ( 'NONE', #10808, #12650, #11141 ) ;
#20713=DIRECTION ( 'NONE',  ( 0.000000000000000000, 1.000000000000000000, -0.000000000000000000 ) ) ;
#20720=DIRECTION ( 'NONE',  ( -1.000000000000000000, 0.000000000000000000, 2.449293598294699019E-16 ) ) ;
#20728=CARTESIAN_POINT ( 'NONE',  ( 163.9999999999998295, 19.17157287525381193, -8.000000000002268408 ) ) ;
#20741=EDGE_CURVE ( 'NONE', #15997, #8292, #11446, .T. ) ;
#20747=ORIENTED_EDGE ( 'NONE', *, *, #2061, .F. ) ;
#20769=DIRECTION ( 'NONE',  ( 0.8981428216242086648, 0.000000000000000000, -0.4397038457472310924 ) ) ;
#20771=LINE ( 'NONE', #1389, #16274 ) ;
#20772=CIRCLE ( 'NONE', #11645, 2.000000000000001776 ) ;
#20775=CARTESIAN_POINT ( 'NONE',  ( 0.000000000000000000, 20.00000000000000000, 0.000000000000000000 ) ) ;
#20782=DIRECTION ( 'NONE',  ( 0.000000000000000000, 1.000000000000000000, 0.000000000000000000 ) ) ;
#20789=EDGE_CURVE ( 'NONE', #1532, #1991, #19951, .T. ) ;
#20809=DIRECTION ( 'NONE',  ( 0.000000000000000000, 0.000000000000000000, 1.000000000000000000 ) ) ;
#20819=ORIENTED_EDGE ( 'NONE', *, *, #6433, .T. ) ;
#20821=ORIENTED_EDGE ( 'NONE', *, *, #18267, .T. ) ;
#20824=CIRCLE ( 'NONE', #11306, 2.000000000000001776 ) ;
#20827=CYLINDRICAL_SURFACE ( 'NONE', #21016, 2.000000000000001776 ) ;
#20832=AXIS2_PLACEMENT_3D ( 'NONE', #15353, #10161, #20720 ) ;
#20835=( BOUNDED_CURVE ( )  B_SPLINE_CURVE ( 3, ( #17788, #9605, #4075, #5791 ),
 .UNSPECIFIED., .F., .T. ) 
 B_SPLINE_CURVE_WITH_KNOTS ( ( 4, 4 ),
 ( 4.712388980384689674, 6.283185307179586232 ),
 .UNSPECIFIED. ) 
 CURVE ( )  GEOMETRIC_REPRESENTATION_ITEM ( )  RATIONAL_B_SPLINE_CURVE ( ( 1.000000000000000000, 0.8047378541243649375, 0.8047378541243649375, 1.000000000000000000 ) ) 
 REPRESENTATION_ITEM ( '' )  );
#20839=CYLINDRICAL_SURFACE ( 'NONE', #18992, 126.0000000000000000 ) ;
#20840=AXIS2_PLACEMENT_3D ( 'NONE', #19911, #756, #5780 ) ;
#20841=EDGE_CURVE ( 'NONE', #11917, #2955, #20147, .T. ) ;
#20842=ORIENTED_EDGE ( 'NONE', *, *, #10996, .T. ) ;
#20846=PLANE ( 'NONE',  #3013 ) ;
#20852=ORIENTED_EDGE ( 'NONE', *, *, #8341, .T. ) ;
#20931=CARTESIAN_POINT ( 'NONE',  ( 0.000000000000000000, 1.999999999999998224, -126.0000000000000000 ) ) ;
#20933=VECTOR ( 'NONE', #17083, 1000.000000000000000 ) ;
#20939=AXIS2_PLACEMENT_3D ( 'NONE', #660, #22293, #1213 ) ;
#20942=CARTESIAN_POINT ( 'NONE',  ( 164.0000000000000000, 20.00000000000000000, 2.250243343269062756E-12 ) ) ;
#20945=FACE_OUTER_BOUND ( 'NONE', #2000, .T. ) ;
#20950=CARTESIAN_POINT ( 'NONE',  ( 0.000000000000000000, 25.00000000000000000, 118.0000000000000000 ) ) ;
#20957=ORIENTED_EDGE ( 'NONE', *, *, #4242, .T. ) ;
#20993=AXIS2_PLACEMENT_3D ( 'NONE', #13093, #22113, #9391 ) ;
#20995=CIRCLE ( 'NONE', #4484, 2.000000000000001776 ) ;
#21002=CARTESIAN_POINT ( 'NONE',  ( 0.000000000000000000, 0.000000000000000000, 124.0000000000000000 ) ) ;
#21014=CARTESIAN_POINT ( 'NONE',  ( 1.028703311283776507E-14, 0.000000000000000000, 83.99999999999998579 ) ) ;
#21016=AXIS2_PLACEMENT_3D ( 'NONE', #8541, #22426, #1339 ) ;
#21019=DIRECTION ( 'NONE',  ( 0.000000000000000000, 1.000000000000000000, 0.000000000000000000 ) ) ;
#21026=AXIS2_PLACEMENT_3D ( 'NONE', #5210, #7393, #17768 ) ;
#21029=EDGE_CURVE ( 'NONE', #11795, #22165, #2247, .T. ) ;
#21031=ORIENTED_EDGE ( 'NONE', *, *, #19692, .T. ) ;
#21035=CARTESIAN_POINT ( 'NONE',  ( 1.469576158976823671E-14, 25.00000000000000000, 120.0000000000000000 ) ) ;
#21038=CARTESIAN_POINT ( 'NONE',  ( -146.5000000000000000, 20.00000000000000000, 10.00000000000002487 ) ) ;
#21044=AXIS2_PLACEMENT_3D ( 'NONE', #4692, #13241, #11725 ) ;
#21048=ORIENTED_EDGE ( 'NONE', *, *, #10556, .T. ) ;
#21077=CARTESIAN_POINT ( 'NONE',  ( -162.0000000000000000, 18.00000000000000355, 53.76161406891260697 ) ) ;
#21084=FACE_BOUND ( 'NONE', #16863, .T. ) ;
#21086=CARTESIAN_POINT ( 'NONE',  ( 1.175660927181459158E-14, 37.00000000000000711, 96.00000000000000000 ) ) ;
#21117=CARTESIAN_POINT ( 'NONE',  ( 9.674709713264089326E-15, 29.00000000000000711, 78.99999999999998579 ) ) ;
#21125=DIRECTION ( 'NONE',  ( 0.8981428216241997831, -0.000000000000000000, 0.4397038457472493556 ) ) ;
#21130=APPLICATION_CONTEXT ( 'automotive_design' ) ;
#21142=ORIENTED_EDGE ( 'NONE', *, *, #9920, .T. ) ;
#21151=EDGE_LOOP ( 'NONE', ( #18146, #9780 ) ) ;
#21165=DIRECTION ( 'NONE',  ( 0.000000000000000000, -1.000000000000000000, 0.000000000000000000 ) ) ;
#21168=ORIENTED_EDGE ( 'NONE', *, *, #5139, .T. ) ;
#21172=CIRCLE ( 'NONE', #4290, 2.000000000000000000 ) ;
#21207=CARTESIAN_POINT ( 'NONE',  ( -164.0000000000000000, 18.00000000000000355, -7.999999999999979572 ) ) ;
#21220=LINE ( 'NONE', #12403, #17362 ) ;
#21232=CARTESIAN_POINT ( 'NONE',  ( 0.000000000000000000, 45.00000000000000000, 110.1134477342067157 ) ) ;
#21251=ORIENTED_EDGE ( 'NONE', *, *, #4338, .F. ) ;
#21266=DIRECTION ( 'NONE',  ( 0.000000000000000000, 0.000000000000000000, 1.000000000000000000 ) ) ;
#21268=VECTOR ( 'NONE', #15308, 1000.000000000000114 ) ;
#21275=ORIENTED_EDGE ( 'NONE', *, *, #18737, .T. ) ;
#21290=ADVANCED_FACE ( 'NONE', ( #7939 ), #6101, .T. ) ;
#21300=ORIENTED_EDGE ( 'NONE', *, *, #22270, .T. ) ;
#21304=EDGE_CURVE ( 'NONE', #21621, #7906, #14001, .T. ) ;
#21311=DIRECTION ( 'NONE',  ( 0.000000000000000000, 0.000000000000000000, 1.000000000000000000 ) ) ;
#21327=AXIS2_PLACEMENT_3D ( 'NONE', #21799, #7927, #14959 ) ;
#21335=CARTESIAN_POINT ( 'NONE',  ( 161.9999999999992610, 20.00000000000000000, -53.76161406891482386 ) ) ;
#21381=EDGE_LOOP ( 'NONE', ( #13729, #15490, #10892, #1401 ) ) ;
#21383=VERTEX_POINT ( 'NONE', #21704 ) ;
#21387=CARTESIAN_POINT ( 'NONE',  ( 146.4999999999998579, 18.00000000000000355, -10.00000000000202860 ) ) ;
#21394=AXIS2_PLACEMENT_3D ( 'NONE', #17465, #13679, #11951 ) ;
#21397=PLANE ( 'NONE',  #8926 ) ;
#21403=CIRCLE ( 'NONE', #14091, 126.0000000000000000 ) ;
#21405=CARTESIAN_POINT ( 'NONE',  ( 55.40268456415108744, 20.00000000000000000, 113.1659955246503557 ) ) ;
#21406=ORIENTED_EDGE ( 'NONE', *, *, #155, .T. ) ;
#21432=ADVANCED_FACE ( 'NONE', ( #17048 ), #8192, .T. ) ;
#21447=CIRCLE ( 'NONE', #16715, 2.000000000000001332 ) ;
#21459=( GEOMETRIC_REPRESENTATION_CONTEXT ( 3 ) GLOBAL_UNCERTAINTY_ASSIGNED_CONTEXT ( ( #272 ) ) GLOBAL_UNIT_ASSIGNED_CONTEXT ( ( #22042, #7838, #11392 ) ) REPRESENTATION_CONTEXT ( 'NONE', 'WORKASPACE' ) );
#21465=LINE ( 'NONE', #927, #19039 ) ;
#21475=CARTESIAN_POINT ( 'NONE',  ( 0.000000000000000000, 18.00000000000000355, 124.0000000000000000 ) ) ;
#21483=DIRECTION ( 'NONE',  ( -0.000000000000000000, -1.000000000000000000, -0.000000000000000000 ) ) ;
#21484=CARTESIAN_POINT ( 'NONE',  ( 0.000000000000000000, 20.00000000000000000, 0.000000000000000000 ) ) ;
#21503=PLANE ( 'NONE',  #7703 ) ;
#21513=ORIENTED_EDGE ( 'NONE', *, *, #16967, .T. ) ;
#21521=CARTESIAN_POINT ( 'NONE',  ( -162.0000000000000000, 20.00000000000000000, 10.00000000000001954 ) ) ;
#21527=DIRECTION ( 'NONE',  ( 0.8981428216242028917, 0.000000000000000000, 0.4397038457472429718 ) ) ;
#21535=CARTESIAN_POINT ( 'NONE',  ( -158.3970384574724619, 2.000000000000000000, -62.74304228515457993 ) ) ;
#21547=VERTEX_POINT ( 'NONE', #3569 ) ;
#21549=ADVANCED_FACE ( 'NONE', ( #1975 ), #12768, .T. ) ;
#21553=ORIENTED_EDGE ( 'NONE', *, *, #2239, .T. ) ;
#21566=ORIENTED_EDGE ( 'NONE', *, *, #2832, .T. ) ;
#21573=EDGE_CURVE ( 'NONE', #6576, #10751, #3906, .T. ) ;
#21595=LINE ( 'NONE', #19883, #18272 ) ;
#21600=AXIS2_PLACEMENT_3D ( 'NONE', #17738, #19867, #19423 ) ;
#21621=VERTEX_POINT ( 'NONE', #1852 ) ;
#21622=ORIENTED_EDGE ( 'NONE', *, *, #11332, .F. ) ;
#21628=AXIS2_PLACEMENT_3D ( 'NONE', #2699, #5773, #977 ) ;
#21629=DIRECTION ( 'NONE',  ( 0.000000000000000000, -1.000000000000000000, 0.000000000000000000 ) ) ;
#21634=ORIENTED_EDGE ( 'NONE', *, *, #20789, .F. ) ;
#21640=CYLINDRICAL_SURFACE ( 'NONE', #5945, 101.0000000000000000 ) ;
#21652=CARTESIAN_POINT ( 'NONE',  ( -164.0000000000000000, 1.999999999999998224, -7.999999999999979572 ) ) ;
#21660=CARTESIAN_POINT ( 'NONE',  ( -1.109343863968193944E-13, 20.00000000000000000, -7.999999999999994671 ) ) ;
#21675=EDGE_CURVE ( 'NONE', #19859, #7803, #2184, .T. ) ;
#21683=VECTOR ( 'NONE', #17848, 1000.000000000000000 ) ;
#21688=FACE_OUTER_BOUND ( 'NONE', #636, .T. ) ;
#21702=CARTESIAN_POINT ( 'NONE',  ( 161.9999999999992610, 1.999999999999998224, 53.76161406891478123 ) ) ;
#21704=CARTESIAN_POINT ( 'NONE',  ( 146.4999999999998863, 18.00000000000000355, -8.000000000002026823 ) ) ;
#21705=EDGE_CURVE ( 'NONE', #19445, #16346, #6675, .T. ) ;
#21729=DIRECTION ( 'NONE',  ( -1.000000000000000000, 0.000000000000000000, -1.387778780781445833E-14 ) ) ;
#21732=CARTESIAN_POINT ( 'NONE',  ( 146.4999999999998863, 1.999999999999998224, 8.000000000001989520 ) ) ;
#21736=DIRECTION ( 'NONE',  ( -0.000000000000000000, -1.000000000000000000, -0.000000000000000000 ) ) ;
#21740=VERTEX_POINT ( 'NONE', #9417 ) ;
#21762=PLANE ( 'NONE',  #2218 ) ;
#21765=ORIENTED_EDGE ( 'NONE', *, *, #18737, .F. ) ;
#21778=ORIENTED_EDGE ( 'NONE', *, *, #1349, .T. ) ;
#21779=CIRCLE ( 'NONE', #9724, 2.000000000000004441 ) ;
#21786=ADVANCED_FACE ( 'NONE', ( #4351 ), #11267, .T. ) ;
#21799=CARTESIAN_POINT ( 'NONE',  ( -9.912705577010314703E-16, 18.00000000000000355, -9.999999999999994671 ) ) ;
#21812=DIRECTION ( 'NONE',  ( -1.000000000000000000, 0.000000000000000000, 1.386679829960243376E-14 ) ) ;
#21817=CYLINDRICAL_SURFACE ( 'NONE', #19714, 2.000000000000001776 ) ;
#21820=CIRCLE ( 'NONE', #11955, 10.00000000000001599 ) ;
#21822=ORIENTED_EDGE ( 'NONE', *, *, #2689, .T. ) ;
#21836=AXIS2_PLACEMENT_3D ( 'NONE', #13683, #5370, #5259 ) ;
#21845=CYLINDRICAL_SURFACE ( 'NONE', #1519, 101.0000000000000000 ) ;
#21858=EDGE_CURVE ( 'NONE', #15773, #21621, #17223, .T. ) ;
#21859=ORIENTED_EDGE ( 'NONE', *, *, #22366, .T. ) ;
#21870=FACE_OUTER_BOUND ( 'NONE', #8464, .T. ) ;
#21875=LINE ( 'NONE', #13319, #3378 ) ;
#21901=LINE ( 'NONE', #13108, #3632 ) ;
#21906=CYLINDRICAL_SURFACE ( 'NONE', #19755, 2.000000000000001776 ) ;
#21907=ADVANCED_FACE ( 'NONE', ( #17022 ), #9977, .T. ) ;
#21918=EDGE_LOOP ( 'NONE', ( #16700, #3862, #2781, #18297 ) ) ;
#21923=ORIENTED_EDGE ( 'NONE', *, *, #13658, .T. ) ;
#21925=FILL_AREA_STYLE ('',( #10014 ) ) ;
#21962=AXIS2_PLACEMENT_3D ( 'NONE', #9405, #16445, #4233 ) ;
#21989=EDGE_LOOP ( 'NONE', ( #13278, #1982, #19393, #15304 ) ) ;
#21996=CARTESIAN_POINT ( 'NONE',  ( -162.0000000000000000, 0.000000000000000000, -9.999999999999978684 ) ) ;
#22021=CARTESIAN_POINT ( 'NONE',  ( 0.000000000000000000, 29.00000000000000711, 0.000000000000000000 ) ) ;
#22037=CARTESIAN_POINT ( 'NONE',  ( -157.5176307659779411, 1.999999999999998224, 60.94675664190624076 ) ) ;
#22039=CARTESIAN_POINT ( 'NONE',  ( -54.52327687265817246, 20.00000000000000000, -111.3697098814011781 ) ) ;
#22042=( LENGTH_UNIT ( ) NAMED_UNIT ( * ) SI_UNIT ( .MILLI., .METRE. ) );
#22044=TOROIDAL_SURFACE ( 'NONE', #1184, 124.0000000000000000, 2.000000000000000000 ) ;
#22079=VECTOR ( 'NONE', #1348, 1000.000000000000000 ) ;
#22090=CYLINDRICAL_SURFACE ( 'NONE', #4379, 2.000000000000000000 ) ;
#22100=ORIENTED_EDGE ( 'NONE', *, *, #6348, .T. ) ;
#22105=EDGE_CURVE ( 'NONE', #18877, #1288, #16925, .T. ) ;
#22106=ORIENTED_EDGE ( 'NONE', *, *, #14591, .F. ) ;
#22113=DIRECTION ( 'NONE',  ( -0.000000000000000000, -1.000000000000000000, 0.000000000000000000 ) ) ;
#22120=DIRECTION ( 'NONE',  ( -0.4397038457472313144, 0.000000000000000000, 0.8981428216242086648 ) ) ;
#22124=AXIS2_PLACEMENT_3D ( 'NONE', #12801, #20011, #9451 ) ;
#22126=FACE_OUTER_BOUND ( 'NONE', #12844, .T. ) ;
#22152=VERTEX_POINT ( 'NONE', #6864 ) ;
#22164=SURFACE_STYLE_FILL_AREA ( #21925 ) ;
#22165=VERTEX_POINT ( 'NONE', #9928 ) ;
#22167=EDGE_CURVE ( 'NONE', #9211, #18877, #12172, .T. ) ;
#22200=DIRECTION ( 'NONE',  ( -0.8981428216242028917, 0.000000000000000000, -0.4397038457472429718 ) ) ;
#22211=DIRECTION ( 'NONE',  ( 0.000000000000000000, 0.000000000000000000, -1.000000000000000000 ) ) ;
#22215=CARTESIAN_POINT ( 'NONE',  ( 0.000000000000000000, 25.00000000000000000, 0.000000000000000000 ) ) ;
#22247=ORIENTED_EDGE ( 'NONE', *, *, #19002, .F. ) ;
#22252=ADVANCED_FACE ( 'NONE', ( #20138 ), #5150, .T. ) ;
#22253=CARTESIAN_POINT ( 'NONE',  ( -154.0000000000000000, 20.00000000000000000, 53.76161406891259986 ) ) ;
#22266=EDGE_LOOP ( 'NONE', ( #2865, #4231, #18242, #3411 ) ) ;
#22267=DIRECTION ( 'NONE',  ( 0.000000000000000000, 1.000000000000000000, -0.000000000000000000 ) ) ;
#22270=EDGE_CURVE ( 'NONE', #8292, #9740, #4731, .T. ) ;
#22282=CARTESIAN_POINT ( 'NONE',  ( -1.362186893977295590E-13, 1.999999999999998224, 9.999999999999994671 ) ) ;
#22293=DIRECTION ( 'NONE',  ( -0.000000000000000000, -1.000000000000000000, 0.000000000000000000 ) ) ;
#22294=CIRCLE ( 'NONE', #6545, 2.000000000000001332 ) ;
#22301=EDGE_CURVE ( 'NONE', #9954, #7572, #11907, .T. ) ;
#22302=VECTOR ( 'NONE', #16485, 1000.000000000000000 ) ;
#22314=CARTESIAN_POINT ( 'NONE',  ( 0.000000000000000000, 0.000000000000000000, 0.000000000000000000 ) ) ;
#22339=DIRECTION ( 'NONE',  ( 1.000000000000000000, 0.000000000000000000, -1.387778780781444413E-14 ) ) ;
#22360=CARTESIAN_POINT ( 'NONE',  ( 163.9999999999998863, 2.000000000000000000, -8.000000000002268408 ) ) ;
#22364=ORIENTED_EDGE ( 'NONE', *, *, #21858, .F. ) ;
#22365=CARTESIAN_POINT ( 'NONE',  ( 161.9999999999992610, 18.00000000000000355, -53.76161406891482386 ) ) ;
#22366=EDGE_CURVE ( 'NONE', #2469, #19973, #11791, .T. ) ;
#22369=CARTESIAN_POINT ( 'NONE',  ( 163.9999999999998863, 1.999999999999998224, -8.000000000002268408 ) ) ;
#22370=DIRECTION ( 'NONE',  ( -0.000000000000000000, -1.000000000000000000, -0.000000000000000000 ) ) ;
#22372=ORIENTED_EDGE ( 'NONE', *, *, #22167, .T. ) ;
#22374=DIRECTION ( 'NONE',  ( 0.8981428216242032248, -6.500054012300580894E-17, -0.4397038457472424167 ) ) ;
#22387=EDGE_CURVE ( 'NONE', #17220, #8554, #2537, .T. ) ;
#22403=CARTESIAN_POINT ( 'NONE',  ( 0.000000000000000000, 23.00000000000000000, 0.000000000000000000 ) ) ;
#22426=DIRECTION ( 'NONE',  ( -1.372099599554306628E-14, 0.000000000000000000, 1.000000000000000000 ) ) ;
#22428=CARTESIAN_POINT ( 'NONE',  ( 54.52327687265658085, 0.000000000000000000, -111.3697098814019171 ) ) ;
#22443=EDGE_LOOP ( 'NONE', ( #10901, #614, #619, #5810, #5543 ) ) ;
#22474=TOROIDAL_SURFACE ( 'NONE', #22124, 118.0000000000000000, 2.000000000000000000 ) ;
#22487=ORIENTED_EDGE ( 'NONE', *, *, #10107, .T. ) ;
#22489=CARTESIAN_POINT ( 'NONE',  ( -90.00000000000000000, 29.00000000000000355, 8.394090934816448357E-16 ) ) ;
#22518=VERTEX_POINT ( 'NONE', #7362 ) ;
#22520=ORIENTED_EDGE ( 'NONE', *, *, #17744, .T. ) ;
#22524=LINE ( 'NONE', #18654, #20321 ) ;
#22532=DIRECTION ( 'NONE',  ( 0.000000000000000000, 1.000000000000000000, 0.000000000000000000 ) ) ;
#22540=DIRECTION ( 'NONE',  ( 0.000000000000000000, 0.000000000000000000, 1.000000000000000000 ) ) ;
#22546=FACE_OUTER_BOUND ( 'NONE', #15767, .T. ) ;
#22562=CARTESIAN_POINT ( 'NONE',  ( 163.9999999999998863, 18.00000000000000355, -8.000000000002268408 ) ) ;
#22577=CARTESIAN_POINT ( 'NONE',  ( -164.0000000000000000, 1.999999999999998224, 8.000000000000019540 ) ) ;
#22583=CARTESIAN_POINT ( 'NONE',  ( -1.432836755002403442E-14, 25.00000000000000000, -117.0000000000000000 ) ) ;
#22587=EDGE_LOOP ( 'NONE', ( #1282, #3809, #2360, #1350 ) ) ;
#22595=ORIENTED_EDGE ( 'NONE', *, *, #8341, .F. ) ;
#22605=CARTESIAN_POINT ( 'NONE',  ( 0.000000000000000000, 18.00000000000000355, -126.0000000000000000 ) ) ;
#22621=DIRECTION ( 'NONE',  ( 1.396592535537253658E-14, -0.000000000000000000, 1.000000000000000000 ) ) ;
#22653=EDGE_CURVE ( 'NONE', #11172, #8011, #17664, .T. ) ;
#22655=EDGE_CURVE ( 'NONE', #15997, #19048, #16220, .T. ) ;
ENDSEC;
END-ISO-10303-21;
